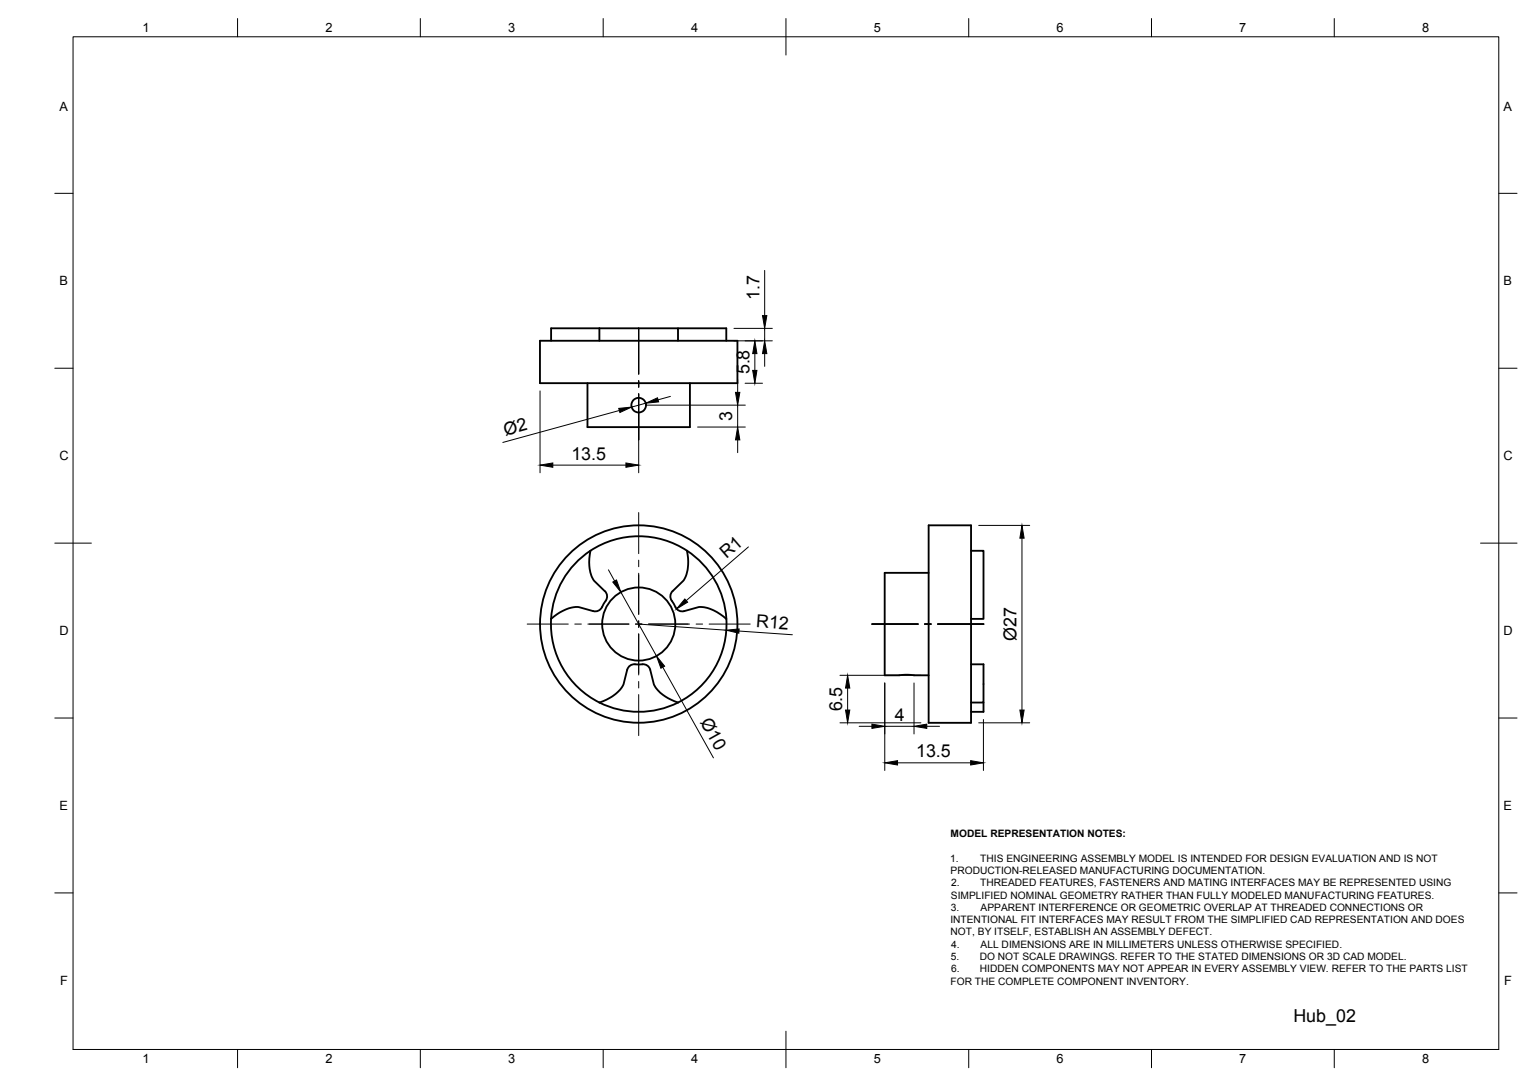
ISO-10303-21;
HEADER;
/* Generated by software containing ST-Developer
 * from STEP Tools, Inc. (www.steptools.com) 
 */

FILE_DESCRIPTION(
/* description */ (''),
/* implementation_level */ '2;1');

FILE_NAME(
/* name */ 'Hub_02.step',
/* time_stamp */ '2026-10-05T21:34:53-07:00',
/* author */ (''),
/* organization */ (''),
/* preprocessor_version */ 'ST-DEVELOPER v20.2',
/* originating_system */ 'Autodesk Translation Framework v15.15.0.0',
/* authorisation */ '');

FILE_SCHEMA (('AUTOMOTIVE_DESIGN { 1 0 10303 214 3 1 1 }'));
ENDSEC;

DATA;
#10=MECHANICAL_DESIGN_GEOMETRIC_PRESENTATION_REPRESENTATION('',(#67),#9822);
#49=SHAPE_REPRESENTATION_RELATIONSHIP('SRR','None',#9859,#58);
#58=ADVANCED_BREP_SHAPE_REPRESENTATION('',(#76),#9815);
#67=STYLED_ITEM('',(#9911),#76);
#76=MANIFOLD_SOLID_BREP('Body1',#3290);
#90=FACE_BOUND('',#562,.T.);
#91=FACE_BOUND('',#566,.T.);
#92=FACE_BOUND('',#568,.T.);
#93=FACE_BOUND('',#570,.T.);
#94=FACE_BOUND('',#573,.T.);
#138=B_SPLINE_CURVE_WITH_KNOTS('',3,(#9018,#9019,#9020,#9021,#9022,#9023,
#9024,#9025,#9026,#9027,#9028,#9029,#9030,#9031,#9032,#9033,#9034,#9035),
 .UNSPECIFIED.,.F.,.F.,(4,2,2,2,2,2,2,2,4),(0.,0.0377244205563716,0.0754488411127431,
0.113172721595804,0.150896602078865,0.188620482561925,0.226344363044986,
0.264068783601358,0.301793204157729),.UNSPECIFIED.);
#139=B_SPLINE_CURVE_WITH_KNOTS('',3,(#9036,#9037,#9038,#9039,#9040,#9041,
#9042,#9043,#9044,#9045,#9046,#9047,#9048,#9049,#9050,#9051,#9052,#9053),
 .UNSPECIFIED.,.F.,.F.,(4,2,2,2,2,2,2,2,4),(0.301793204157729,0.339517624714101,
0.377242045270472,0.414965925753533,0.452689806236594,0.490413686719655,
0.528137567202715,0.565861987759087,0.603586408315459),.UNSPECIFIED.);
#140=B_SPLINE_CURVE_WITH_KNOTS('',3,(#9074,#9075,#9076,#9077,#9078,#9079,
#9080,#9081,#9082,#9083,#9084,#9085,#9086,#9087,#9088,#9089,#9090,#9091),
 .UNSPECIFIED.,.F.,.F.,(4,2,2,2,2,2,2,2,4),(-0.302227736861757,-0.264448211272738,
-0.226668685683718,-0.188891277057298,-0.151113868430879,-0.113336459804459,
-0.0755590511780388,-0.0377795255890194,0.),.UNSPECIFIED.);
#141=B_SPLINE_CURVE_WITH_KNOTS('',3,(#9151,#9152,#9153,#9154,#9155,#9156,
#9157,#9158,#9159,#9160),.UNSPECIFIED.,.F.,.F.,(4,2,2,2,4),(-0.142515337525874,
-0.116550796129695,-0.0827833358062311,-0.0239794870259187,0.),
 .UNSPECIFIED.);
#142=B_SPLINE_CURVE_WITH_KNOTS('',3,(#9171,#9172,#9173,#9174,#9175,#9176,
#9177,#9178,#9179,#9180),.UNSPECIFIED.,.F.,.F.,(4,2,2,2,4),(-1.69587031053129,
-0.72373117069956,-0.441822634924292,-0.252830368936358,0.),
 .UNSPECIFIED.);
#143=B_SPLINE_CURVE_WITH_KNOTS('',3,(#9182,#9183,#9184,#9185,#9186,#9187,
#9188,#9189,#9190,#9191),.UNSPECIFIED.,.F.,.F.,(4,2,2,2,4),(-0.142515337583282,
-0.116550796158019,-0.0827833358058086,-0.0239794870257561,0.),
 .UNSPECIFIED.);
#144=B_SPLINE_CURVE_WITH_KNOTS('',3,(#9202,#9203,#9204,#9205,#9206,#9207,
#9208,#9209,#9210,#9211),.UNSPECIFIED.,.F.,.F.,(4,2,2,2,4),(-1.69587031141743,
-0.723731170975569,-0.441822635061051,-0.252830368989318,0.),
 .UNSPECIFIED.);
#145=B_SPLINE_CURVE_WITH_KNOTS('',3,(#9213,#9214,#9215,#9216,#9217,#9218,
#9219,#9220,#9221,#9222),.UNSPECIFIED.,.F.,.F.,(4,2,2,2,4),(-0.142515337540036,
-0.116550796137795,-0.0827833358078941,-0.0239794870259568,0.),
 .UNSPECIFIED.);
#146=B_SPLINE_CURVE_WITH_KNOTS('',3,(#9233,#9234,#9235,#9236,#9237,#9238,
#9239,#9240,#9241,#9242),.UNSPECIFIED.,.F.,.F.,(4,2,2,2,4),(-1.69587030996743,
-0.72373117051105,-0.441822634822492,-0.252830368895713,0.),
 .UNSPECIFIED.);
#147=B_SPLINE_CURVE_WITH_KNOTS('',3,(#9289,#9290,#9291,#9292,#9293,#9294,
#9295,#9296,#9297,#9298),.UNSPECIFIED.,.F.,.F.,(4,2,2,2,4),(-0.142515337540036,
-0.116550796137795,-0.0827833358078941,-0.0239794870259568,0.),
 .UNSPECIFIED.);
#148=B_SPLINE_CURVE_WITH_KNOTS('',3,(#9321,#9322,#9323,#9324,#9325,#9326,
#9327,#9328,#9329,#9330),.UNSPECIFIED.,.F.,.F.,(4,2,2,2,4),(-1.69587030996743,
-0.72373117051105,-0.441822634822492,-0.252830368895713,0.),
 .UNSPECIFIED.);
#149=B_SPLINE_CURVE_WITH_KNOTS('',3,(#9372,#9373,#9374,#9375,#9376,#9377,
#9378,#9379,#9380,#9381),.UNSPECIFIED.,.F.,.F.,(4,2,2,2,4),(-0.142515337583282,
-0.116550796158019,-0.0827833358058086,-0.0239794870257561,0.),
 .UNSPECIFIED.);
#150=B_SPLINE_CURVE_WITH_KNOTS('',3,(#9404,#9405,#9406,#9407,#9408,#9409,
#9410,#9411,#9412,#9413),.UNSPECIFIED.,.F.,.F.,(4,2,2,2,4),(-1.69587031141743,
-0.723731170975569,-0.441822635061051,-0.252830368989318,0.),
 .UNSPECIFIED.);
#151=B_SPLINE_CURVE_WITH_KNOTS('',3,(#9457,#9458,#9459,#9460,#9461,#9462,
#9463,#9464,#9465,#9466),.UNSPECIFIED.,.F.,.F.,(4,2,2,2,4),(-0.142515337525874,
-0.116550796129695,-0.0827833358062311,-0.0239794870259187,0.),
 .UNSPECIFIED.);
#152=B_SPLINE_CURVE_WITH_KNOTS('',3,(#9493,#9494,#9495,#9496,#9497,#9498,
#9499,#9500,#9501,#9502),.UNSPECIFIED.,.F.,.F.,(4,2,2,2,4),(-1.69587031053129,
-0.72373117069956,-0.441822634924292,-0.252830368936358,0.),
 .UNSPECIFIED.);
#175=B_SPLINE_SURFACE_WITH_KNOTS('',3,1,((#9269,#9270),(#9271,#9272),(#9273,
#9274),(#9275,#9276),(#9277,#9278),(#9279,#9280),(#9281,#9282),(#9283,#9284),
(#9285,#9286),(#9287,#9288)),.UNSPECIFIED.,.F.,.F.,.F.,(4,2,2,2,4),(2,2),
(-0.142515337540036,-0.116550796137795,-0.0827833358078941,-0.0239794870259568,
0.),(0.,0.78),.UNSPECIFIED.);
#176=B_SPLINE_SURFACE_WITH_KNOTS('',3,1,((#9299,#9300),(#9301,#9302),(#9303,
#9304),(#9305,#9306),(#9307,#9308),(#9309,#9310),(#9311,#9312),(#9313,#9314),
(#9315,#9316),(#9317,#9318)),.UNSPECIFIED.,.F.,.F.,.F.,(4,2,2,2,4),(2,2),
(-1.69587030996743,-0.72373117051105,-0.441822634822492,-0.252830368895713,
0.),(0.,0.78),.UNSPECIFIED.);
#177=B_SPLINE_SURFACE_WITH_KNOTS('',3,1,((#9352,#9353),(#9354,#9355),(#9356,
#9357),(#9358,#9359),(#9360,#9361),(#9362,#9363),(#9364,#9365),(#9366,#9367),
(#9368,#9369),(#9370,#9371)),.UNSPECIFIED.,.F.,.F.,.F.,(4,2,2,2,4),(2,2),
(-0.142515337583282,-0.116550796158019,-0.0827833358058086,-0.0239794870257561,
0.),(0.,0.78),.UNSPECIFIED.);
#178=B_SPLINE_SURFACE_WITH_KNOTS('',3,1,((#9382,#9383),(#9384,#9385),(#9386,
#9387),(#9388,#9389),(#9390,#9391),(#9392,#9393),(#9394,#9395),(#9396,#9397),
(#9398,#9399),(#9400,#9401)),.UNSPECIFIED.,.F.,.F.,.F.,(4,2,2,2,4),(2,2),
(-1.69587031141743,-0.723731170975569,-0.441822635061051,-0.252830368989318,
0.),(0.,0.78),.UNSPECIFIED.);
#179=B_SPLINE_SURFACE_WITH_KNOTS('',3,1,((#9435,#9436),(#9437,#9438),(#9439,
#9440),(#9441,#9442),(#9443,#9444),(#9445,#9446),(#9447,#9448),(#9449,#9450),
(#9451,#9452),(#9453,#9454)),.UNSPECIFIED.,.F.,.F.,.F.,(4,2,2,2,4),(2,2),
(-0.142515337525874,-0.116550796129695,-0.0827833358062311,-0.0239794870259187,
0.),(0.,0.78),.UNSPECIFIED.);
#180=B_SPLINE_SURFACE_WITH_KNOTS('',3,1,((#9471,#9472),(#9473,#9474),(#9475,
#9476),(#9477,#9478),(#9479,#9480),(#9481,#9482),(#9483,#9484),(#9485,#9486),
(#9487,#9488),(#9489,#9490)),.UNSPECIFIED.,.F.,.F.,.F.,(4,2,2,2,4),(2,2),
(-1.69587031053129,-0.72373117069956,-0.441822634924292,-0.252830368936358,
0.),(0.,0.78),.UNSPECIFIED.);
#212=PLANE('',#3570);
#213=PLANE('',#3571);
#214=PLANE('',#3573);
#215=PLANE('',#3575);
#216=PLANE('',#3589);
#217=PLANE('',#3598);
#218=PLANE('',#3611);
#219=PLANE('',#3614);
#220=PLANE('',#3619);
#221=PLANE('',#3620);
#222=PLANE('',#3623);
#223=PLANE('',#3628);
#224=PLANE('',#3629);
#225=PLANE('',#3632);
#226=PLANE('',#3637);
#227=PLANE('',#3640);
#228=PLANE('',#3643);
#359=FACE_OUTER_BOUND('',#551,.T.);
#360=FACE_OUTER_BOUND('',#552,.T.);
#361=FACE_OUTER_BOUND('',#553,.T.);
#362=FACE_OUTER_BOUND('',#554,.T.);
#363=FACE_OUTER_BOUND('',#555,.T.);
#364=FACE_OUTER_BOUND('',#556,.T.);
#365=FACE_OUTER_BOUND('',#557,.T.);
#366=FACE_OUTER_BOUND('',#558,.T.);
#367=FACE_OUTER_BOUND('',#559,.T.);
#368=FACE_OUTER_BOUND('',#560,.T.);
#369=FACE_OUTER_BOUND('',#561,.T.);
#370=FACE_OUTER_BOUND('',#563,.T.);
#371=FACE_OUTER_BOUND('',#564,.T.);
#372=FACE_OUTER_BOUND('',#565,.T.);
#373=FACE_OUTER_BOUND('',#567,.T.);
#374=FACE_OUTER_BOUND('',#569,.T.);
#375=FACE_OUTER_BOUND('',#571,.T.);
#376=FACE_OUTER_BOUND('',#572,.T.);
#377=FACE_OUTER_BOUND('',#574,.T.);
#378=FACE_OUTER_BOUND('',#575,.T.);
#379=FACE_OUTER_BOUND('',#576,.T.);
#380=FACE_OUTER_BOUND('',#577,.T.);
#381=FACE_OUTER_BOUND('',#578,.T.);
#382=FACE_OUTER_BOUND('',#579,.T.);
#383=FACE_OUTER_BOUND('',#580,.T.);
#384=FACE_OUTER_BOUND('',#581,.T.);
#385=FACE_OUTER_BOUND('',#582,.T.);
#386=FACE_OUTER_BOUND('',#583,.T.);
#387=FACE_OUTER_BOUND('',#584,.T.);
#388=FACE_OUTER_BOUND('',#585,.T.);
#389=FACE_OUTER_BOUND('',#586,.T.);
#390=FACE_OUTER_BOUND('',#587,.T.);
#391=FACE_OUTER_BOUND('',#588,.T.);
#392=FACE_OUTER_BOUND('',#589,.T.);
#393=FACE_OUTER_BOUND('',#590,.T.);
#394=FACE_OUTER_BOUND('',#591,.T.);
#395=FACE_OUTER_BOUND('',#592,.T.);
#396=FACE_OUTER_BOUND('',#593,.T.);
#397=FACE_OUTER_BOUND('',#594,.T.);
#398=FACE_OUTER_BOUND('',#595,.T.);
#399=FACE_OUTER_BOUND('',#596,.T.);
#400=FACE_OUTER_BOUND('',#597,.T.);
#401=FACE_OUTER_BOUND('',#598,.T.);
#551=EDGE_LOOP('',(#2610,#2611,#2612,#2613,#2614,#2615));
#552=EDGE_LOOP('',(#2616,#2617,#2618,#2619));
#553=EDGE_LOOP('',(#2620,#2621,#2622,#2623));
#554=EDGE_LOOP('',(#2624,#2625,#2626,#2627,#2628));
#555=EDGE_LOOP('',(#2629,#2630,#2631,#2632));
#556=EDGE_LOOP('',(#2633,#2634,#2635,#2636,#2637));
#557=EDGE_LOOP('',(#2638,#2639,#2640,#2641,#2642,#2643,#2644,#2645));
#558=EDGE_LOOP('',(#2646,#2647,#2648,#2649));
#559=EDGE_LOOP('',(#2650,#2651,#2652,#2653));
#560=EDGE_LOOP('',(#2654,#2655,#2656,#2657));
#561=EDGE_LOOP('',(#2658));
#562=EDGE_LOOP('',(#2659,#2660,#2661,#2662,#2663,#2664));
#563=EDGE_LOOP('',(#2665,#2666,#2667,#2668));
#564=EDGE_LOOP('',(#2669,#2670,#2671,#2672));
#565=EDGE_LOOP('',(#2673,#2674,#2675,#2676,#2677,#2678,#2679,#2680,#2681,
#2682,#2683,#2684,#2685,#2686,#2687,#2688,#2689,#2690,#2691,#2692,#2693,
#2694,#2695,#2696));
#566=EDGE_LOOP('',(#2697));
#567=EDGE_LOOP('',(#2698,#2699,#2700,#2701));
#568=EDGE_LOOP('',(#2702,#2703));
#569=EDGE_LOOP('',(#2704));
#570=EDGE_LOOP('',(#2705,#2706,#2707,#2708,#2709));
#571=EDGE_LOOP('',(#2710,#2711,#2712,#2713));
#572=EDGE_LOOP('',(#2714));
#573=EDGE_LOOP('',(#2715));
#574=EDGE_LOOP('',(#2716,#2717,#2718,#2719));
#575=EDGE_LOOP('',(#2720,#2721,#2722,#2723));
#576=EDGE_LOOP('',(#2724,#2725,#2726,#2727));
#577=EDGE_LOOP('',(#2728,#2729,#2730,#2731,#2732));
#578=EDGE_LOOP('',(#2733,#2734,#2735,#2736,#2737));
#579=EDGE_LOOP('',(#2738,#2739,#2740,#2741));
#580=EDGE_LOOP('',(#2742,#2743,#2744,#2745));
#581=EDGE_LOOP('',(#2746,#2747,#2748,#2749,#2750,#2751,#2752,#2753));
#582=EDGE_LOOP('',(#2754,#2755,#2756,#2757));
#583=EDGE_LOOP('',(#2758,#2759,#2760,#2761));
#584=EDGE_LOOP('',(#2762,#2763,#2764,#2765));
#585=EDGE_LOOP('',(#2766,#2767,#2768,#2769,#2770));
#586=EDGE_LOOP('',(#2771,#2772,#2773,#2774,#2775));
#587=EDGE_LOOP('',(#2776,#2777,#2778,#2779));
#588=EDGE_LOOP('',(#2780,#2781,#2782,#2783));
#589=EDGE_LOOP('',(#2784,#2785,#2786,#2787,#2788,#2789,#2790,#2791));
#590=EDGE_LOOP('',(#2792,#2793,#2794,#2795));
#591=EDGE_LOOP('',(#2796,#2797,#2798,#2799));
#592=EDGE_LOOP('',(#2800,#2801,#2802,#2803));
#593=EDGE_LOOP('',(#2804,#2805,#2806,#2807,#2808));
#594=EDGE_LOOP('',(#2809,#2810,#2811,#2812));
#595=EDGE_LOOP('',(#2813,#2814,#2815,#2816,#2817));
#596=EDGE_LOOP('',(#2818,#2819,#2820,#2821));
#597=EDGE_LOOP('',(#2822,#2823,#2824,#2825));
#598=EDGE_LOOP('',(#2826,#2827,#2828,#2829,#2830,#2831,#2832,#2833));
#781=LINE('',#9016,#1040);
#782=LINE('',#9056,#1041);
#783=LINE('',#9058,#1042);
#784=LINE('',#9059,#1043);
#785=LINE('',#9062,#1044);
#786=LINE('',#9065,#1045);
#787=LINE('',#9068,#1046);
#788=LINE('',#9070,#1047);
#789=LINE('',#9071,#1048);
#790=LINE('',#9092,#1049);
#791=LINE('',#9095,#1050);
#792=LINE('',#9096,#1051);
#793=LINE('',#9101,#1052);
#794=LINE('',#9107,#1053);
#795=LINE('',#9111,#1054);
#796=LINE('',#9116,#1055);
#797=LINE('',#9120,#1056);
#798=LINE('',#9125,#1057);
#799=LINE('',#9129,#1058);
#800=LINE('',#9139,#1059);
#801=LINE('',#9142,#1060);
#802=LINE('',#9145,#1061);
#803=LINE('',#9148,#1062);
#804=LINE('',#9162,#1063);
#805=LINE('',#9170,#1064);
#806=LINE('',#9193,#1065);
#807=LINE('',#9201,#1066);
#808=LINE('',#9224,#1067);
#809=LINE('',#9232,#1068);
#810=LINE('',#9247,#1069);
#811=LINE('',#9252,#1070);
#812=LINE('',#9257,#1071);
#813=LINE('',#9260,#1072);
#814=LINE('',#9263,#1073);
#815=LINE('',#9267,#1074);
#816=LINE('',#9268,#1075);
#817=LINE('',#9320,#1076);
#818=LINE('',#9333,#1077);
#819=LINE('',#9334,#1078);
#820=LINE('',#9340,#1079);
#821=LINE('',#9343,#1080);
#822=LINE('',#9346,#1081);
#823=LINE('',#9350,#1082);
#824=LINE('',#9351,#1083);
#825=LINE('',#9403,#1084);
#826=LINE('',#9416,#1085);
#827=LINE('',#9417,#1086);
#828=LINE('',#9423,#1087);
#829=LINE('',#9426,#1088);
#830=LINE('',#9429,#1089);
#831=LINE('',#9433,#1090);
#832=LINE('',#9434,#1091);
#833=LINE('',#9456,#1092);
#834=LINE('',#9469,#1093);
#835=LINE('',#9492,#1094);
#836=LINE('',#9505,#1095);
#837=LINE('',#9506,#1096);
#1040=VECTOR('',#4203,1.);
#1041=VECTOR('',#4206,10.);
#1042=VECTOR('',#4207,10.);
#1043=VECTOR('',#4208,10.);
#1044=VECTOR('',#4211,10.);
#1045=VECTOR('',#4214,10.);
#1046=VECTOR('',#4217,10.);
#1047=VECTOR('',#4218,10.);
#1048=VECTOR('',#4219,10.);
#1049=VECTOR('',#4222,10.);
#1050=VECTOR('',#4225,10.);
#1051=VECTOR('',#4226,10.);
#1052=VECTOR('',#4231,5.);
#1053=VECTOR('',#4238,10.);
#1054=VECTOR('',#4241,10.);
#1055=VECTOR('',#4246,10.);
#1056=VECTOR('',#4249,10.);
#1057=VECTOR('',#4254,10.);
#1058=VECTOR('',#4257,10.);
#1059=VECTOR('',#4272,10.);
#1060=VECTOR('',#4275,10.);
#1061=VECTOR('',#4278,10.);
#1062=VECTOR('',#4281,10.);
#1063=VECTOR('',#4284,10.);
#1064=VECTOR('',#4291,10.);
#1065=VECTOR('',#4292,10.);
#1066=VECTOR('',#4299,10.);
#1067=VECTOR('',#4300,10.);
#1068=VECTOR('',#4307,10.);
#1069=VECTOR('',#4312,7.);
#1070=VECTOR('',#4319,13.5);
#1071=VECTOR('',#4326,10.);
#1072=VECTOR('',#4329,10.);
#1073=VECTOR('',#4332,10.);
#1074=VECTOR('',#4337,10.);
#1075=VECTOR('',#4338,10.);
#1076=VECTOR('',#4339,10.);
#1077=VECTOR('',#4342,10.);
#1078=VECTOR('',#4343,10.);
#1079=VECTOR('',#4352,10.);
#1080=VECTOR('',#4355,10.);
#1081=VECTOR('',#4358,10.);
#1082=VECTOR('',#4363,10.);
#1083=VECTOR('',#4364,10.);
#1084=VECTOR('',#4365,10.);
#1085=VECTOR('',#4368,10.);
#1086=VECTOR('',#4369,10.);
#1087=VECTOR('',#4378,10.);
#1088=VECTOR('',#4381,10.);
#1089=VECTOR('',#4384,10.);
#1090=VECTOR('',#4389,10.);
#1091=VECTOR('',#4390,10.);
#1092=VECTOR('',#4391,10.);
#1093=VECTOR('',#4394,10.);
#1094=VECTOR('',#4397,10.);
#1095=VECTOR('',#4400,10.);
#1096=VECTOR('',#4401,10.);
#1259=CIRCLE('',#3568,1.);
#1260=CIRCLE('',#3569,1.);
#1261=CIRCLE('',#3572,1.);
#1262=CIRCLE('',#3577,5.);
#1263=CIRCLE('',#3578,5.);
#1264=CIRCLE('',#3579,5.);
#1265=CIRCLE('',#3581,12.);
#1266=CIRCLE('',#3582,12.);
#1267=CIRCLE('',#3584,12.);
#1268=CIRCLE('',#3585,12.);
#1269=CIRCLE('',#3587,12.);
#1270=CIRCLE('',#3588,12.);
#1271=CIRCLE('',#3590,13.5);
#1272=CIRCLE('',#3591,12.);
#1273=CIRCLE('',#3592,12.);
#1274=CIRCLE('',#3593,12.);
#1275=CIRCLE('',#3595,12.);
#1276=CIRCLE('',#3597,12.);
#1277=CIRCLE('',#3599,1.);
#1278=CIRCLE('',#3600,5.529);
#1279=CIRCLE('',#3601,1.);
#1280=CIRCLE('',#3602,1.);
#1281=CIRCLE('',#3603,5.529);
#1282=CIRCLE('',#3604,1.);
#1283=CIRCLE('',#3605,1.);
#1284=CIRCLE('',#3606,5.529);
#1285=CIRCLE('',#3607,1.);
#1286=CIRCLE('',#3609,7.);
#1287=CIRCLE('',#3610,7.);
#1288=CIRCLE('',#3613,13.5);
#1289=CIRCLE('',#3616,5.529);
#1290=CIRCLE('',#3618,1.);
#1291=CIRCLE('',#3622,1.);
#1292=CIRCLE('',#3625,5.529);
#1293=CIRCLE('',#3627,1.);
#1294=CIRCLE('',#3631,1.);
#1295=CIRCLE('',#3634,5.529);
#1296=CIRCLE('',#3636,1.);
#1297=CIRCLE('',#3639,12.);
#1298=CIRCLE('',#3642,1.);
#1489=VERTEX_POINT('',#9011);
#1490=VERTEX_POINT('',#9012);
#1491=VERTEX_POINT('',#9015);
#1492=VERTEX_POINT('',#9017);
#1493=VERTEX_POINT('',#9055);
#1494=VERTEX_POINT('',#9057);
#1495=VERTEX_POINT('',#9061);
#1496=VERTEX_POINT('',#9063);
#1497=VERTEX_POINT('',#9067);
#1498=VERTEX_POINT('',#9069);
#1499=VERTEX_POINT('',#9073);
#1500=VERTEX_POINT('',#9094);
#1501=VERTEX_POINT('',#9098);
#1502=VERTEX_POINT('',#9100);
#1503=VERTEX_POINT('',#9105);
#1504=VERTEX_POINT('',#9106);
#1505=VERTEX_POINT('',#9108);
#1506=VERTEX_POINT('',#9110);
#1507=VERTEX_POINT('',#9114);
#1508=VERTEX_POINT('',#9115);
#1509=VERTEX_POINT('',#9117);
#1510=VERTEX_POINT('',#9119);
#1511=VERTEX_POINT('',#9123);
#1512=VERTEX_POINT('',#9124);
#1513=VERTEX_POINT('',#9126);
#1514=VERTEX_POINT('',#9128);
#1515=VERTEX_POINT('',#9132);
#1516=VERTEX_POINT('',#9138);
#1517=VERTEX_POINT('',#9140);
#1518=VERTEX_POINT('',#9144);
#1519=VERTEX_POINT('',#9146);
#1520=VERTEX_POINT('',#9150);
#1521=VERTEX_POINT('',#9161);
#1522=VERTEX_POINT('',#9163);
#1523=VERTEX_POINT('',#9165);
#1524=VERTEX_POINT('',#9167);
#1525=VERTEX_POINT('',#9169);
#1526=VERTEX_POINT('',#9181);
#1527=VERTEX_POINT('',#9192);
#1528=VERTEX_POINT('',#9194);
#1529=VERTEX_POINT('',#9196);
#1530=VERTEX_POINT('',#9198);
#1531=VERTEX_POINT('',#9200);
#1532=VERTEX_POINT('',#9212);
#1533=VERTEX_POINT('',#9223);
#1534=VERTEX_POINT('',#9225);
#1535=VERTEX_POINT('',#9227);
#1536=VERTEX_POINT('',#9229);
#1537=VERTEX_POINT('',#9231);
#1538=VERTEX_POINT('',#9244);
#1539=VERTEX_POINT('',#9246);
#1540=VERTEX_POINT('',#9251);
#1541=VERTEX_POINT('',#9256);
#1542=VERTEX_POINT('',#9258);
#1543=VERTEX_POINT('',#9262);
#1544=VERTEX_POINT('',#9266);
#1545=VERTEX_POINT('',#9319);
#1546=VERTEX_POINT('',#9332);
#1547=VERTEX_POINT('',#9339);
#1548=VERTEX_POINT('',#9341);
#1549=VERTEX_POINT('',#9345);
#1550=VERTEX_POINT('',#9349);
#1551=VERTEX_POINT('',#9402);
#1552=VERTEX_POINT('',#9415);
#1553=VERTEX_POINT('',#9422);
#1554=VERTEX_POINT('',#9424);
#1555=VERTEX_POINT('',#9428);
#1556=VERTEX_POINT('',#9432);
#1557=VERTEX_POINT('',#9455);
#1558=VERTEX_POINT('',#9468);
#1559=VERTEX_POINT('',#9491);
#1560=VERTEX_POINT('',#9504);
#1884=EDGE_CURVE('',#1489,#1490,#1259,.T.);
#1885=EDGE_CURVE('',#1490,#1489,#1260,.T.);
#1886=EDGE_CURVE('',#1490,#1491,#781,.T.);
#1887=EDGE_CURVE('',#1492,#1491,#138,.T.);
#1888=EDGE_CURVE('',#1491,#1492,#139,.T.);
#1889=EDGE_CURVE('',#1489,#1493,#782,.T.);
#1890=EDGE_CURVE('',#1494,#1493,#783,.T.);
#1891=EDGE_CURVE('',#1494,#1490,#784,.T.);
#1892=EDGE_CURVE('',#1490,#1495,#785,.T.);
#1893=EDGE_CURVE('',#1495,#1496,#1261,.T.);
#1894=EDGE_CURVE('',#1496,#1489,#786,.T.);
#1895=EDGE_CURVE('',#1493,#1497,#787,.T.);
#1896=EDGE_CURVE('',#1498,#1496,#788,.T.);
#1897=EDGE_CURVE('',#1497,#1498,#789,.T.);
#1898=EDGE_CURVE('',#1498,#1499,#140,.T.);
#1899=EDGE_CURVE('',#1499,#1495,#790,.T.);
#1900=EDGE_CURVE('',#1500,#1494,#791,.T.);
#1901=EDGE_CURVE('',#1499,#1500,#792,.T.);
#1902=EDGE_CURVE('',#1500,#1501,#1262,.T.);
#1903=EDGE_CURVE('',#1501,#1502,#793,.T.);
#1904=EDGE_CURVE('',#1502,#1502,#1263,.T.);
#1905=EDGE_CURVE('',#1501,#1497,#1264,.T.);
#1906=EDGE_CURVE('',#1503,#1504,#794,.T.);
#1907=EDGE_CURVE('',#1504,#1505,#1265,.T.);
#1908=EDGE_CURVE('',#1506,#1505,#795,.T.);
#1909=EDGE_CURVE('',#1506,#1503,#1266,.T.);
#1910=EDGE_CURVE('',#1507,#1508,#796,.T.);
#1911=EDGE_CURVE('',#1507,#1509,#1267,.T.);
#1912=EDGE_CURVE('',#1509,#1510,#797,.T.);
#1913=EDGE_CURVE('',#1510,#1508,#1268,.T.);
#1914=EDGE_CURVE('',#1511,#1512,#798,.T.);
#1915=EDGE_CURVE('',#1511,#1513,#1269,.T.);
#1916=EDGE_CURVE('',#1513,#1514,#799,.T.);
#1917=EDGE_CURVE('',#1514,#1512,#1270,.T.);
#1918=EDGE_CURVE('',#1515,#1515,#1271,.T.);
#1919=EDGE_CURVE('',#1514,#1508,#1272,.T.);
#1920=EDGE_CURVE('',#1510,#1505,#1273,.T.);
#1921=EDGE_CURVE('',#1504,#1512,#1274,.T.);
#1922=EDGE_CURVE('',#1514,#1516,#800,.T.);
#1923=EDGE_CURVE('',#1516,#1517,#1275,.T.);
#1924=EDGE_CURVE('',#1508,#1517,#801,.T.);
#1925=EDGE_CURVE('',#1510,#1518,#802,.T.);
#1926=EDGE_CURVE('',#1518,#1519,#1276,.T.);
#1927=EDGE_CURVE('',#1505,#1519,#803,.T.);
#1928=EDGE_CURVE('',#1511,#1520,#141,.T.);
#1929=EDGE_CURVE('',#1520,#1521,#804,.T.);
#1930=EDGE_CURVE('',#1522,#1521,#1277,.T.);
#1931=EDGE_CURVE('',#1522,#1523,#1278,.T.);
#1932=EDGE_CURVE('',#1524,#1523,#1279,.T.);
#1933=EDGE_CURVE('',#1524,#1525,#805,.T.);
#1934=EDGE_CURVE('',#1525,#1503,#142,.T.);
#1935=EDGE_CURVE('',#1506,#1526,#143,.T.);
#1936=EDGE_CURVE('',#1526,#1527,#806,.T.);
#1937=EDGE_CURVE('',#1528,#1527,#1280,.T.);
#1938=EDGE_CURVE('',#1528,#1529,#1281,.T.);
#1939=EDGE_CURVE('',#1530,#1529,#1282,.T.);
#1940=EDGE_CURVE('',#1530,#1531,#807,.T.);
#1941=EDGE_CURVE('',#1531,#1509,#144,.T.);
#1942=EDGE_CURVE('',#1507,#1532,#145,.T.);
#1943=EDGE_CURVE('',#1532,#1533,#808,.T.);
#1944=EDGE_CURVE('',#1534,#1533,#1283,.T.);
#1945=EDGE_CURVE('',#1534,#1535,#1284,.T.);
#1946=EDGE_CURVE('',#1536,#1535,#1285,.T.);
#1947=EDGE_CURVE('',#1536,#1537,#809,.T.);
#1948=EDGE_CURVE('',#1537,#1513,#146,.T.);
#1949=EDGE_CURVE('',#1538,#1538,#1286,.F.);
#1950=EDGE_CURVE('',#1538,#1539,#810,.T.);
#1951=EDGE_CURVE('',#1539,#1539,#1287,.T.);
#1952=EDGE_CURVE('',#1515,#1540,#811,.T.);
#1953=EDGE_CURVE('',#1540,#1540,#1288,.T.);
#1954=EDGE_CURVE('',#1534,#1541,#812,.T.);
#1955=EDGE_CURVE('',#1541,#1542,#1289,.T.);
#1956=EDGE_CURVE('',#1535,#1542,#813,.T.);
#1957=EDGE_CURVE('',#1533,#1543,#814,.T.);
#1958=EDGE_CURVE('',#1543,#1541,#1290,.T.);
#1959=EDGE_CURVE('',#1532,#1544,#815,.T.);
#1960=EDGE_CURVE('',#1544,#1543,#816,.T.);
#1961=EDGE_CURVE('',#1517,#1544,#147,.T.);
#1962=EDGE_CURVE('',#1537,#1545,#817,.T.);
#1963=EDGE_CURVE('',#1545,#1516,#148,.T.);
#1964=EDGE_CURVE('',#1536,#1546,#818,.T.);
#1965=EDGE_CURVE('',#1546,#1545,#819,.T.);
#1966=EDGE_CURVE('',#1542,#1546,#1291,.T.);
#1967=EDGE_CURVE('',#1528,#1547,#820,.T.);
#1968=EDGE_CURVE('',#1547,#1548,#1292,.T.);
#1969=EDGE_CURVE('',#1529,#1548,#821,.T.);
#1970=EDGE_CURVE('',#1527,#1549,#822,.T.);
#1971=EDGE_CURVE('',#1549,#1547,#1293,.T.);
#1972=EDGE_CURVE('',#1526,#1550,#823,.T.);
#1973=EDGE_CURVE('',#1550,#1549,#824,.T.);
#1974=EDGE_CURVE('',#1519,#1550,#149,.T.);
#1975=EDGE_CURVE('',#1531,#1551,#825,.T.);
#1976=EDGE_CURVE('',#1551,#1518,#150,.T.);
#1977=EDGE_CURVE('',#1530,#1552,#826,.T.);
#1978=EDGE_CURVE('',#1552,#1551,#827,.T.);
#1979=EDGE_CURVE('',#1548,#1552,#1294,.T.);
#1980=EDGE_CURVE('',#1522,#1553,#828,.T.);
#1981=EDGE_CURVE('',#1553,#1554,#1295,.T.);
#1982=EDGE_CURVE('',#1523,#1554,#829,.T.);
#1983=EDGE_CURVE('',#1521,#1555,#830,.T.);
#1984=EDGE_CURVE('',#1555,#1553,#1296,.T.);
#1985=EDGE_CURVE('',#1520,#1556,#831,.T.);
#1986=EDGE_CURVE('',#1556,#1555,#832,.T.);
#1987=EDGE_CURVE('',#1512,#1557,#833,.T.);
#1988=EDGE_CURVE('',#1557,#1556,#151,.T.);
#1989=EDGE_CURVE('',#1504,#1558,#834,.T.);
#1990=EDGE_CURVE('',#1558,#1557,#1297,.T.);
#1991=EDGE_CURVE('',#1525,#1559,#835,.T.);
#1992=EDGE_CURVE('',#1559,#1558,#152,.T.);
#1993=EDGE_CURVE('',#1524,#1560,#836,.T.);
#1994=EDGE_CURVE('',#1560,#1559,#837,.T.);
#1995=EDGE_CURVE('',#1554,#1560,#1298,.T.);
#2610=ORIENTED_EDGE('',*,*,#1884,.F.);
#2611=ORIENTED_EDGE('',*,*,#1885,.F.);
#2612=ORIENTED_EDGE('',*,*,#1886,.T.);
#2613=ORIENTED_EDGE('',*,*,#1887,.F.);
#2614=ORIENTED_EDGE('',*,*,#1888,.F.);
#2615=ORIENTED_EDGE('',*,*,#1886,.F.);
#2616=ORIENTED_EDGE('',*,*,#1885,.T.);
#2617=ORIENTED_EDGE('',*,*,#1889,.T.);
#2618=ORIENTED_EDGE('',*,*,#1890,.F.);
#2619=ORIENTED_EDGE('',*,*,#1891,.T.);
#2620=ORIENTED_EDGE('',*,*,#1884,.T.);
#2621=ORIENTED_EDGE('',*,*,#1892,.T.);
#2622=ORIENTED_EDGE('',*,*,#1893,.T.);
#2623=ORIENTED_EDGE('',*,*,#1894,.T.);
#2624=ORIENTED_EDGE('',*,*,#1895,.F.);
#2625=ORIENTED_EDGE('',*,*,#1889,.F.);
#2626=ORIENTED_EDGE('',*,*,#1894,.F.);
#2627=ORIENTED_EDGE('',*,*,#1896,.F.);
#2628=ORIENTED_EDGE('',*,*,#1897,.F.);
#2629=ORIENTED_EDGE('',*,*,#1898,.F.);
#2630=ORIENTED_EDGE('',*,*,#1896,.T.);
#2631=ORIENTED_EDGE('',*,*,#1893,.F.);
#2632=ORIENTED_EDGE('',*,*,#1899,.F.);
#2633=ORIENTED_EDGE('',*,*,#1900,.F.);
#2634=ORIENTED_EDGE('',*,*,#1901,.F.);
#2635=ORIENTED_EDGE('',*,*,#1899,.T.);
#2636=ORIENTED_EDGE('',*,*,#1892,.F.);
#2637=ORIENTED_EDGE('',*,*,#1891,.F.);
#2638=ORIENTED_EDGE('',*,*,#1902,.T.);
#2639=ORIENTED_EDGE('',*,*,#1903,.T.);
#2640=ORIENTED_EDGE('',*,*,#1904,.F.);
#2641=ORIENTED_EDGE('',*,*,#1903,.F.);
#2642=ORIENTED_EDGE('',*,*,#1905,.T.);
#2643=ORIENTED_EDGE('',*,*,#1897,.T.);
#2644=ORIENTED_EDGE('',*,*,#1898,.T.);
#2645=ORIENTED_EDGE('',*,*,#1901,.T.);
#2646=ORIENTED_EDGE('',*,*,#1906,.T.);
#2647=ORIENTED_EDGE('',*,*,#1907,.T.);
#2648=ORIENTED_EDGE('',*,*,#1908,.F.);
#2649=ORIENTED_EDGE('',*,*,#1909,.T.);
#2650=ORIENTED_EDGE('',*,*,#1910,.F.);
#2651=ORIENTED_EDGE('',*,*,#1911,.T.);
#2652=ORIENTED_EDGE('',*,*,#1912,.T.);
#2653=ORIENTED_EDGE('',*,*,#1913,.T.);
#2654=ORIENTED_EDGE('',*,*,#1914,.F.);
#2655=ORIENTED_EDGE('',*,*,#1915,.T.);
#2656=ORIENTED_EDGE('',*,*,#1916,.T.);
#2657=ORIENTED_EDGE('',*,*,#1917,.T.);
#2658=ORIENTED_EDGE('',*,*,#1918,.F.);
#2659=ORIENTED_EDGE('',*,*,#1919,.T.);
#2660=ORIENTED_EDGE('',*,*,#1913,.F.);
#2661=ORIENTED_EDGE('',*,*,#1920,.T.);
#2662=ORIENTED_EDGE('',*,*,#1907,.F.);
#2663=ORIENTED_EDGE('',*,*,#1921,.T.);
#2664=ORIENTED_EDGE('',*,*,#1917,.F.);
#2665=ORIENTED_EDGE('',*,*,#1919,.F.);
#2666=ORIENTED_EDGE('',*,*,#1922,.T.);
#2667=ORIENTED_EDGE('',*,*,#1923,.T.);
#2668=ORIENTED_EDGE('',*,*,#1924,.F.);
#2669=ORIENTED_EDGE('',*,*,#1920,.F.);
#2670=ORIENTED_EDGE('',*,*,#1925,.T.);
#2671=ORIENTED_EDGE('',*,*,#1926,.T.);
#2672=ORIENTED_EDGE('',*,*,#1927,.F.);
#2673=ORIENTED_EDGE('',*,*,#1915,.F.);
#2674=ORIENTED_EDGE('',*,*,#1928,.T.);
#2675=ORIENTED_EDGE('',*,*,#1929,.T.);
#2676=ORIENTED_EDGE('',*,*,#1930,.F.);
#2677=ORIENTED_EDGE('',*,*,#1931,.T.);
#2678=ORIENTED_EDGE('',*,*,#1932,.F.);
#2679=ORIENTED_EDGE('',*,*,#1933,.T.);
#2680=ORIENTED_EDGE('',*,*,#1934,.T.);
#2681=ORIENTED_EDGE('',*,*,#1909,.F.);
#2682=ORIENTED_EDGE('',*,*,#1935,.T.);
#2683=ORIENTED_EDGE('',*,*,#1936,.T.);
#2684=ORIENTED_EDGE('',*,*,#1937,.F.);
#2685=ORIENTED_EDGE('',*,*,#1938,.T.);
#2686=ORIENTED_EDGE('',*,*,#1939,.F.);
#2687=ORIENTED_EDGE('',*,*,#1940,.T.);
#2688=ORIENTED_EDGE('',*,*,#1941,.T.);
#2689=ORIENTED_EDGE('',*,*,#1911,.F.);
#2690=ORIENTED_EDGE('',*,*,#1942,.T.);
#2691=ORIENTED_EDGE('',*,*,#1943,.T.);
#2692=ORIENTED_EDGE('',*,*,#1944,.F.);
#2693=ORIENTED_EDGE('',*,*,#1945,.T.);
#2694=ORIENTED_EDGE('',*,*,#1946,.F.);
#2695=ORIENTED_EDGE('',*,*,#1947,.T.);
#2696=ORIENTED_EDGE('',*,*,#1948,.T.);
#2697=ORIENTED_EDGE('',*,*,#1904,.T.);
#2698=ORIENTED_EDGE('',*,*,#1949,.T.);
#2699=ORIENTED_EDGE('',*,*,#1950,.T.);
#2700=ORIENTED_EDGE('',*,*,#1951,.T.);
#2701=ORIENTED_EDGE('',*,*,#1950,.F.);
#2702=ORIENTED_EDGE('',*,*,#1887,.T.);
#2703=ORIENTED_EDGE('',*,*,#1888,.T.);
#2704=ORIENTED_EDGE('',*,*,#1951,.F.);
#2705=ORIENTED_EDGE('',*,*,#1895,.T.);
#2706=ORIENTED_EDGE('',*,*,#1905,.F.);
#2707=ORIENTED_EDGE('',*,*,#1902,.F.);
#2708=ORIENTED_EDGE('',*,*,#1900,.T.);
#2709=ORIENTED_EDGE('',*,*,#1890,.T.);
#2710=ORIENTED_EDGE('',*,*,#1918,.T.);
#2711=ORIENTED_EDGE('',*,*,#1952,.T.);
#2712=ORIENTED_EDGE('',*,*,#1953,.T.);
#2713=ORIENTED_EDGE('',*,*,#1952,.F.);
#2714=ORIENTED_EDGE('',*,*,#1953,.F.);
#2715=ORIENTED_EDGE('',*,*,#1949,.F.);
#2716=ORIENTED_EDGE('',*,*,#1945,.F.);
#2717=ORIENTED_EDGE('',*,*,#1954,.T.);
#2718=ORIENTED_EDGE('',*,*,#1955,.T.);
#2719=ORIENTED_EDGE('',*,*,#1956,.F.);
#2720=ORIENTED_EDGE('',*,*,#1944,.T.);
#2721=ORIENTED_EDGE('',*,*,#1957,.T.);
#2722=ORIENTED_EDGE('',*,*,#1958,.T.);
#2723=ORIENTED_EDGE('',*,*,#1954,.F.);
#2724=ORIENTED_EDGE('',*,*,#1943,.F.);
#2725=ORIENTED_EDGE('',*,*,#1959,.T.);
#2726=ORIENTED_EDGE('',*,*,#1960,.T.);
#2727=ORIENTED_EDGE('',*,*,#1957,.F.);
#2728=ORIENTED_EDGE('',*,*,#1942,.F.);
#2729=ORIENTED_EDGE('',*,*,#1910,.T.);
#2730=ORIENTED_EDGE('',*,*,#1924,.T.);
#2731=ORIENTED_EDGE('',*,*,#1961,.T.);
#2732=ORIENTED_EDGE('',*,*,#1959,.F.);
#2733=ORIENTED_EDGE('',*,*,#1948,.F.);
#2734=ORIENTED_EDGE('',*,*,#1962,.T.);
#2735=ORIENTED_EDGE('',*,*,#1963,.T.);
#2736=ORIENTED_EDGE('',*,*,#1922,.F.);
#2737=ORIENTED_EDGE('',*,*,#1916,.F.);
#2738=ORIENTED_EDGE('',*,*,#1947,.F.);
#2739=ORIENTED_EDGE('',*,*,#1964,.T.);
#2740=ORIENTED_EDGE('',*,*,#1965,.T.);
#2741=ORIENTED_EDGE('',*,*,#1962,.F.);
#2742=ORIENTED_EDGE('',*,*,#1946,.T.);
#2743=ORIENTED_EDGE('',*,*,#1956,.T.);
#2744=ORIENTED_EDGE('',*,*,#1966,.T.);
#2745=ORIENTED_EDGE('',*,*,#1964,.F.);
#2746=ORIENTED_EDGE('',*,*,#1966,.F.);
#2747=ORIENTED_EDGE('',*,*,#1955,.F.);
#2748=ORIENTED_EDGE('',*,*,#1958,.F.);
#2749=ORIENTED_EDGE('',*,*,#1960,.F.);
#2750=ORIENTED_EDGE('',*,*,#1961,.F.);
#2751=ORIENTED_EDGE('',*,*,#1923,.F.);
#2752=ORIENTED_EDGE('',*,*,#1963,.F.);
#2753=ORIENTED_EDGE('',*,*,#1965,.F.);
#2754=ORIENTED_EDGE('',*,*,#1938,.F.);
#2755=ORIENTED_EDGE('',*,*,#1967,.T.);
#2756=ORIENTED_EDGE('',*,*,#1968,.T.);
#2757=ORIENTED_EDGE('',*,*,#1969,.F.);
#2758=ORIENTED_EDGE('',*,*,#1937,.T.);
#2759=ORIENTED_EDGE('',*,*,#1970,.T.);
#2760=ORIENTED_EDGE('',*,*,#1971,.T.);
#2761=ORIENTED_EDGE('',*,*,#1967,.F.);
#2762=ORIENTED_EDGE('',*,*,#1936,.F.);
#2763=ORIENTED_EDGE('',*,*,#1972,.T.);
#2764=ORIENTED_EDGE('',*,*,#1973,.T.);
#2765=ORIENTED_EDGE('',*,*,#1970,.F.);
#2766=ORIENTED_EDGE('',*,*,#1935,.F.);
#2767=ORIENTED_EDGE('',*,*,#1908,.T.);
#2768=ORIENTED_EDGE('',*,*,#1927,.T.);
#2769=ORIENTED_EDGE('',*,*,#1974,.T.);
#2770=ORIENTED_EDGE('',*,*,#1972,.F.);
#2771=ORIENTED_EDGE('',*,*,#1941,.F.);
#2772=ORIENTED_EDGE('',*,*,#1975,.T.);
#2773=ORIENTED_EDGE('',*,*,#1976,.T.);
#2774=ORIENTED_EDGE('',*,*,#1925,.F.);
#2775=ORIENTED_EDGE('',*,*,#1912,.F.);
#2776=ORIENTED_EDGE('',*,*,#1940,.F.);
#2777=ORIENTED_EDGE('',*,*,#1977,.T.);
#2778=ORIENTED_EDGE('',*,*,#1978,.T.);
#2779=ORIENTED_EDGE('',*,*,#1975,.F.);
#2780=ORIENTED_EDGE('',*,*,#1939,.T.);
#2781=ORIENTED_EDGE('',*,*,#1969,.T.);
#2782=ORIENTED_EDGE('',*,*,#1979,.T.);
#2783=ORIENTED_EDGE('',*,*,#1977,.F.);
#2784=ORIENTED_EDGE('',*,*,#1979,.F.);
#2785=ORIENTED_EDGE('',*,*,#1968,.F.);
#2786=ORIENTED_EDGE('',*,*,#1971,.F.);
#2787=ORIENTED_EDGE('',*,*,#1973,.F.);
#2788=ORIENTED_EDGE('',*,*,#1974,.F.);
#2789=ORIENTED_EDGE('',*,*,#1926,.F.);
#2790=ORIENTED_EDGE('',*,*,#1976,.F.);
#2791=ORIENTED_EDGE('',*,*,#1978,.F.);
#2792=ORIENTED_EDGE('',*,*,#1931,.F.);
#2793=ORIENTED_EDGE('',*,*,#1980,.T.);
#2794=ORIENTED_EDGE('',*,*,#1981,.T.);
#2795=ORIENTED_EDGE('',*,*,#1982,.F.);
#2796=ORIENTED_EDGE('',*,*,#1930,.T.);
#2797=ORIENTED_EDGE('',*,*,#1983,.T.);
#2798=ORIENTED_EDGE('',*,*,#1984,.T.);
#2799=ORIENTED_EDGE('',*,*,#1980,.F.);
#2800=ORIENTED_EDGE('',*,*,#1929,.F.);
#2801=ORIENTED_EDGE('',*,*,#1985,.T.);
#2802=ORIENTED_EDGE('',*,*,#1986,.T.);
#2803=ORIENTED_EDGE('',*,*,#1983,.F.);
#2804=ORIENTED_EDGE('',*,*,#1928,.F.);
#2805=ORIENTED_EDGE('',*,*,#1914,.T.);
#2806=ORIENTED_EDGE('',*,*,#1987,.T.);
#2807=ORIENTED_EDGE('',*,*,#1988,.T.);
#2808=ORIENTED_EDGE('',*,*,#1985,.F.);
#2809=ORIENTED_EDGE('',*,*,#1921,.F.);
#2810=ORIENTED_EDGE('',*,*,#1989,.T.);
#2811=ORIENTED_EDGE('',*,*,#1990,.T.);
#2812=ORIENTED_EDGE('',*,*,#1987,.F.);
#2813=ORIENTED_EDGE('',*,*,#1934,.F.);
#2814=ORIENTED_EDGE('',*,*,#1991,.T.);
#2815=ORIENTED_EDGE('',*,*,#1992,.T.);
#2816=ORIENTED_EDGE('',*,*,#1989,.F.);
#2817=ORIENTED_EDGE('',*,*,#1906,.F.);
#2818=ORIENTED_EDGE('',*,*,#1933,.F.);
#2819=ORIENTED_EDGE('',*,*,#1993,.T.);
#2820=ORIENTED_EDGE('',*,*,#1994,.T.);
#2821=ORIENTED_EDGE('',*,*,#1991,.F.);
#2822=ORIENTED_EDGE('',*,*,#1932,.T.);
#2823=ORIENTED_EDGE('',*,*,#1982,.T.);
#2824=ORIENTED_EDGE('',*,*,#1995,.T.);
#2825=ORIENTED_EDGE('',*,*,#1993,.F.);
#2826=ORIENTED_EDGE('',*,*,#1995,.F.);
#2827=ORIENTED_EDGE('',*,*,#1981,.F.);
#2828=ORIENTED_EDGE('',*,*,#1984,.F.);
#2829=ORIENTED_EDGE('',*,*,#1986,.F.);
#2830=ORIENTED_EDGE('',*,*,#1988,.F.);
#2831=ORIENTED_EDGE('',*,*,#1990,.F.);
#2832=ORIENTED_EDGE('',*,*,#1992,.F.);
#2833=ORIENTED_EDGE('',*,*,#1994,.F.);
#3071=CYLINDRICAL_SURFACE('',#3567,1.);
#3072=CYLINDRICAL_SURFACE('',#3574,1.);
#3073=CYLINDRICAL_SURFACE('',#3576,5.);
#3074=CYLINDRICAL_SURFACE('',#3580,12.);
#3075=CYLINDRICAL_SURFACE('',#3583,12.);
#3076=CYLINDRICAL_SURFACE('',#3586,12.);
#3077=CYLINDRICAL_SURFACE('',#3594,12.);
#3078=CYLINDRICAL_SURFACE('',#3596,12.);
#3079=CYLINDRICAL_SURFACE('',#3608,7.);
#3080=CYLINDRICAL_SURFACE('',#3612,13.5);
#3081=CYLINDRICAL_SURFACE('',#3615,5.529);
#3082=CYLINDRICAL_SURFACE('',#3617,1.);
#3083=CYLINDRICAL_SURFACE('',#3621,1.);
#3084=CYLINDRICAL_SURFACE('',#3624,5.529);
#3085=CYLINDRICAL_SURFACE('',#3626,1.);
#3086=CYLINDRICAL_SURFACE('',#3630,1.);
#3087=CYLINDRICAL_SURFACE('',#3633,5.529);
#3088=CYLINDRICAL_SURFACE('',#3635,1.);
#3089=CYLINDRICAL_SURFACE('',#3638,12.);
#3090=CYLINDRICAL_SURFACE('',#3641,1.);
#3197=ADVANCED_FACE('',(#359),#3071,.F.);
#3198=ADVANCED_FACE('',(#360),#212,.F.);
#3199=ADVANCED_FACE('',(#361),#213,.F.);
#3200=ADVANCED_FACE('',(#362),#214,.T.);
#3201=ADVANCED_FACE('',(#363),#3072,.F.);
#3202=ADVANCED_FACE('',(#364),#215,.T.);
#3203=ADVANCED_FACE('',(#365),#3073,.F.);
#3204=ADVANCED_FACE('',(#366),#3074,.F.);
#3205=ADVANCED_FACE('',(#367),#3075,.F.);
#3206=ADVANCED_FACE('',(#368),#3076,.F.);
#3207=ADVANCED_FACE('',(#369,#90),#216,.T.);
#3208=ADVANCED_FACE('',(#370),#3077,.T.);
#3209=ADVANCED_FACE('',(#371),#3078,.T.);
#3210=ADVANCED_FACE('',(#372,#91),#217,.T.);
#3211=ADVANCED_FACE('',(#373,#92),#3079,.T.);
#3212=ADVANCED_FACE('',(#374,#93),#218,.F.);
#3213=ADVANCED_FACE('',(#375),#3080,.T.);
#3214=ADVANCED_FACE('',(#376,#94),#219,.F.);
#3215=ADVANCED_FACE('',(#377),#3081,.F.);
#3216=ADVANCED_FACE('',(#378),#3082,.T.);
#3217=ADVANCED_FACE('',(#379),#220,.F.);
#3218=ADVANCED_FACE('',(#380),#175,.F.);
#3219=ADVANCED_FACE('',(#381),#176,.F.);
#3220=ADVANCED_FACE('',(#382),#221,.F.);
#3221=ADVANCED_FACE('',(#383),#3083,.T.);
#3222=ADVANCED_FACE('',(#384),#222,.T.);
#3223=ADVANCED_FACE('',(#385),#3084,.F.);
#3224=ADVANCED_FACE('',(#386),#3085,.T.);
#3225=ADVANCED_FACE('',(#387),#223,.F.);
#3226=ADVANCED_FACE('',(#388),#177,.F.);
#3227=ADVANCED_FACE('',(#389),#178,.F.);
#3228=ADVANCED_FACE('',(#390),#224,.F.);
#3229=ADVANCED_FACE('',(#391),#3086,.T.);
#3230=ADVANCED_FACE('',(#392),#225,.T.);
#3231=ADVANCED_FACE('',(#393),#3087,.F.);
#3232=ADVANCED_FACE('',(#394),#3088,.T.);
#3233=ADVANCED_FACE('',(#395),#226,.F.);
#3234=ADVANCED_FACE('',(#396),#179,.F.);
#3235=ADVANCED_FACE('',(#397),#3089,.T.);
#3236=ADVANCED_FACE('',(#398),#180,.F.);
#3237=ADVANCED_FACE('',(#399),#227,.F.);
#3238=ADVANCED_FACE('',(#400),#3090,.T.);
#3239=ADVANCED_FACE('',(#401),#228,.T.);
#3290=CLOSED_SHELL('',(#3197,#3198,#3199,#3200,#3201,#3202,#3203,#3204,
#3205,#3206,#3207,#3208,#3209,#3210,#3211,#3212,#3213,#3214,#3215,#3216,
#3217,#3218,#3219,#3220,#3221,#3222,#3223,#3224,#3225,#3226,#3227,#3228,
#3229,#3230,#3231,#3232,#3233,#3234,#3235,#3236,#3237,#3238,#3239));
#3566=AXIS2_PLACEMENT_3D('',#9009,#4195,#4196);
#3567=AXIS2_PLACEMENT_3D('',#9010,#4197,#4198);
#3568=AXIS2_PLACEMENT_3D('',#9013,#4199,#4200);
#3569=AXIS2_PLACEMENT_3D('',#9014,#4201,#4202);
#3570=AXIS2_PLACEMENT_3D('',#9054,#4204,#4205);
#3571=AXIS2_PLACEMENT_3D('',#9060,#4209,#4210);
#3572=AXIS2_PLACEMENT_3D('',#9064,#4212,#4213);
#3573=AXIS2_PLACEMENT_3D('',#9066,#4215,#4216);
#3574=AXIS2_PLACEMENT_3D('',#9072,#4220,#4221);
#3575=AXIS2_PLACEMENT_3D('',#9093,#4223,#4224);
#3576=AXIS2_PLACEMENT_3D('',#9097,#4227,#4228);
#3577=AXIS2_PLACEMENT_3D('',#9099,#4229,#4230);
#3578=AXIS2_PLACEMENT_3D('',#9102,#4232,#4233);
#3579=AXIS2_PLACEMENT_3D('',#9103,#4234,#4235);
#3580=AXIS2_PLACEMENT_3D('',#9104,#4236,#4237);
#3581=AXIS2_PLACEMENT_3D('',#9109,#4239,#4240);
#3582=AXIS2_PLACEMENT_3D('',#9112,#4242,#4243);
#3583=AXIS2_PLACEMENT_3D('',#9113,#4244,#4245);
#3584=AXIS2_PLACEMENT_3D('',#9118,#4247,#4248);
#3585=AXIS2_PLACEMENT_3D('',#9121,#4250,#4251);
#3586=AXIS2_PLACEMENT_3D('',#9122,#4252,#4253);
#3587=AXIS2_PLACEMENT_3D('',#9127,#4255,#4256);
#3588=AXIS2_PLACEMENT_3D('',#9130,#4258,#4259);
#3589=AXIS2_PLACEMENT_3D('',#9131,#4260,#4261);
#3590=AXIS2_PLACEMENT_3D('',#9133,#4262,#4263);
#3591=AXIS2_PLACEMENT_3D('',#9134,#4264,#4265);
#3592=AXIS2_PLACEMENT_3D('',#9135,#4266,#4267);
#3593=AXIS2_PLACEMENT_3D('',#9136,#4268,#4269);
#3594=AXIS2_PLACEMENT_3D('',#9137,#4270,#4271);
#3595=AXIS2_PLACEMENT_3D('',#9141,#4273,#4274);
#3596=AXIS2_PLACEMENT_3D('',#9143,#4276,#4277);
#3597=AXIS2_PLACEMENT_3D('',#9147,#4279,#4280);
#3598=AXIS2_PLACEMENT_3D('',#9149,#4282,#4283);
#3599=AXIS2_PLACEMENT_3D('',#9164,#4285,#4286);
#3600=AXIS2_PLACEMENT_3D('',#9166,#4287,#4288);
#3601=AXIS2_PLACEMENT_3D('',#9168,#4289,#4290);
#3602=AXIS2_PLACEMENT_3D('',#9195,#4293,#4294);
#3603=AXIS2_PLACEMENT_3D('',#9197,#4295,#4296);
#3604=AXIS2_PLACEMENT_3D('',#9199,#4297,#4298);
#3605=AXIS2_PLACEMENT_3D('',#9226,#4301,#4302);
#3606=AXIS2_PLACEMENT_3D('',#9228,#4303,#4304);
#3607=AXIS2_PLACEMENT_3D('',#9230,#4305,#4306);
#3608=AXIS2_PLACEMENT_3D('',#9243,#4308,#4309);
#3609=AXIS2_PLACEMENT_3D('',#9245,#4310,#4311);
#3610=AXIS2_PLACEMENT_3D('',#9248,#4313,#4314);
#3611=AXIS2_PLACEMENT_3D('',#9249,#4315,#4316);
#3612=AXIS2_PLACEMENT_3D('',#9250,#4317,#4318);
#3613=AXIS2_PLACEMENT_3D('',#9253,#4320,#4321);
#3614=AXIS2_PLACEMENT_3D('',#9254,#4322,#4323);
#3615=AXIS2_PLACEMENT_3D('',#9255,#4324,#4325);
#3616=AXIS2_PLACEMENT_3D('',#9259,#4327,#4328);
#3617=AXIS2_PLACEMENT_3D('',#9261,#4330,#4331);
#3618=AXIS2_PLACEMENT_3D('',#9264,#4333,#4334);
#3619=AXIS2_PLACEMENT_3D('',#9265,#4335,#4336);
#3620=AXIS2_PLACEMENT_3D('',#9331,#4340,#4341);
#3621=AXIS2_PLACEMENT_3D('',#9335,#4344,#4345);
#3622=AXIS2_PLACEMENT_3D('',#9336,#4346,#4347);
#3623=AXIS2_PLACEMENT_3D('',#9337,#4348,#4349);
#3624=AXIS2_PLACEMENT_3D('',#9338,#4350,#4351);
#3625=AXIS2_PLACEMENT_3D('',#9342,#4353,#4354);
#3626=AXIS2_PLACEMENT_3D('',#9344,#4356,#4357);
#3627=AXIS2_PLACEMENT_3D('',#9347,#4359,#4360);
#3628=AXIS2_PLACEMENT_3D('',#9348,#4361,#4362);
#3629=AXIS2_PLACEMENT_3D('',#9414,#4366,#4367);
#3630=AXIS2_PLACEMENT_3D('',#9418,#4370,#4371);
#3631=AXIS2_PLACEMENT_3D('',#9419,#4372,#4373);
#3632=AXIS2_PLACEMENT_3D('',#9420,#4374,#4375);
#3633=AXIS2_PLACEMENT_3D('',#9421,#4376,#4377);
#3634=AXIS2_PLACEMENT_3D('',#9425,#4379,#4380);
#3635=AXIS2_PLACEMENT_3D('',#9427,#4382,#4383);
#3636=AXIS2_PLACEMENT_3D('',#9430,#4385,#4386);
#3637=AXIS2_PLACEMENT_3D('',#9431,#4387,#4388);
#3638=AXIS2_PLACEMENT_3D('',#9467,#4392,#4393);
#3639=AXIS2_PLACEMENT_3D('',#9470,#4395,#4396);
#3640=AXIS2_PLACEMENT_3D('',#9503,#4398,#4399);
#3641=AXIS2_PLACEMENT_3D('',#9507,#4402,#4403);
#3642=AXIS2_PLACEMENT_3D('',#9508,#4404,#4405);
#3643=AXIS2_PLACEMENT_3D('',#9509,#4406,#4407);
#4195=DIRECTION('axis',(0.,0.,1.));
#4196=DIRECTION('refdir',(1.,0.,0.));
#4197=DIRECTION('center_axis',(0.,-1.,0.));
#4198=DIRECTION('ref_axis',(1.,0.,0.));
#4199=DIRECTION('center_axis',(0.,-1.,0.));
#4200=DIRECTION('ref_axis',(1.,0.,0.));
#4201=DIRECTION('center_axis',(0.,-1.,0.));
#4202=DIRECTION('ref_axis',(1.,0.,0.));
#4203=DIRECTION('',(0.,-1.,0.));
#4204=DIRECTION('center_axis',(0.,-1.,0.));
#4205=DIRECTION('ref_axis',(1.,0.,0.));
#4206=DIRECTION('',(0.,0.,-1.));
#4207=DIRECTION('',(1.,0.,0.));
#4208=DIRECTION('',(0.,0.,1.));
#4209=DIRECTION('center_axis',(0.,-1.,0.));
#4210=DIRECTION('ref_axis',(1.,0.,0.));
#4211=DIRECTION('',(0.,0.,1.));
#4212=DIRECTION('center_axis',(0.,1.,0.));
#4213=DIRECTION('ref_axis',(1.,0.,0.));
#4214=DIRECTION('',(0.,0.,-1.));
#4215=DIRECTION('center_axis',(-1.,0.,0.));
#4216=DIRECTION('ref_axis',(0.,0.,-1.));
#4217=DIRECTION('',(0.,1.,0.));
#4218=DIRECTION('',(0.,-1.,0.));
#4219=DIRECTION('',(0.,0.,1.));
#4220=DIRECTION('center_axis',(0.,1.,0.));
#4221=DIRECTION('ref_axis',(1.,0.,0.));
#4222=DIRECTION('',(0.,-1.,0.));
#4223=DIRECTION('center_axis',(1.,0.,0.));
#4224=DIRECTION('ref_axis',(0.,0.,1.));
#4225=DIRECTION('',(0.,-1.,0.));
#4226=DIRECTION('',(0.,0.,-1.));
#4227=DIRECTION('center_axis',(0.,0.,1.));
#4228=DIRECTION('ref_axis',(0.5,-0.866025403784439,0.));
#4229=DIRECTION('center_axis',(0.,0.,-1.));
#4230=DIRECTION('ref_axis',(-0.5,0.866025403784439,0.));
#4231=DIRECTION('',(0.,0.,1.));
#4232=DIRECTION('center_axis',(0.,0.,-1.));
#4233=DIRECTION('ref_axis',(0.5,-0.866025403784439,0.));
#4234=DIRECTION('center_axis',(0.,0.,-1.));
#4235=DIRECTION('ref_axis',(-0.5,0.866025403784439,0.));
#4236=DIRECTION('center_axis',(0.,0.,-1.));
#4237=DIRECTION('ref_axis',(0.5,-0.866025403784439,0.));
#4238=DIRECTION('',(0.,0.,1.));
#4239=DIRECTION('center_axis',(0.,0.,1.));
#4240=DIRECTION('ref_axis',(0.5,-0.866025403784439,0.));
#4241=DIRECTION('',(0.,0.,1.));
#4242=DIRECTION('center_axis',(0.,0.,-1.));
#4243=DIRECTION('ref_axis',(0.5,-0.866025403784439,0.));
#4244=DIRECTION('center_axis',(0.,0.,-1.));
#4245=DIRECTION('ref_axis',(0.,1.,0.));
#4246=DIRECTION('',(0.,0.,1.));
#4247=DIRECTION('center_axis',(0.,0.,-1.));
#4248=DIRECTION('ref_axis',(0.5,-0.866025403784439,0.));
#4249=DIRECTION('',(0.,0.,1.));
#4250=DIRECTION('center_axis',(0.,0.,1.));
#4251=DIRECTION('ref_axis',(0.5,-0.866025403784439,0.));
#4252=DIRECTION('center_axis',(0.,0.,-1.));
#4253=DIRECTION('ref_axis',(0.5,-0.866025403784439,0.));
#4254=DIRECTION('',(0.,0.,1.));
#4255=DIRECTION('center_axis',(0.,0.,-1.));
#4256=DIRECTION('ref_axis',(0.5,-0.866025403784439,0.));
#4257=DIRECTION('',(0.,0.,1.));
#4258=DIRECTION('center_axis',(0.,0.,1.));
#4259=DIRECTION('ref_axis',(0.5,-0.866025403784439,0.));
#4260=DIRECTION('center_axis',(0.,0.,1.));
#4261=DIRECTION('ref_axis',(0.5,-0.866025403784439,0.));
#4262=DIRECTION('center_axis',(0.,0.,-1.));
#4263=DIRECTION('ref_axis',(0.5,-0.866025403784439,0.));
#4264=DIRECTION('center_axis',(0.,0.,-1.));
#4265=DIRECTION('ref_axis',(0.5,-0.866025403784439,0.));
#4266=DIRECTION('center_axis',(0.,0.,-1.));
#4267=DIRECTION('ref_axis',(0.5,-0.866025403784439,0.));
#4268=DIRECTION('center_axis',(0.,0.,-1.));
#4269=DIRECTION('ref_axis',(0.5,-0.866025403784439,0.));
#4270=DIRECTION('center_axis',(0.,0.,-1.));
#4271=DIRECTION('ref_axis',(0.5,-0.866025403784439,0.));
#4272=DIRECTION('',(0.,0.,1.));
#4273=DIRECTION('center_axis',(0.,0.,-1.));
#4274=DIRECTION('ref_axis',(0.5,-0.866025403784439,0.));
#4275=DIRECTION('',(0.,0.,1.));
#4276=DIRECTION('center_axis',(0.,0.,-1.));
#4277=DIRECTION('ref_axis',(0.5,-0.866025403784439,0.));
#4278=DIRECTION('',(0.,0.,1.));
#4279=DIRECTION('center_axis',(0.,0.,-1.));
#4280=DIRECTION('ref_axis',(0.5,-0.866025403784439,0.));
#4281=DIRECTION('',(0.,0.,1.));
#4282=DIRECTION('center_axis',(0.,0.,1.));
#4283=DIRECTION('ref_axis',(0.5,-0.866025403784439,0.));
#4284=DIRECTION('',(0.244394302218901,0.969675938158175,0.));
#4285=DIRECTION('center_axis',(0.,0.,1.));
#4286=DIRECTION('ref_axis',(0.092992392522802,0.995666819238687,0.));
#4287=DIRECTION('center_axis',(0.,0.,1.));
#4288=DIRECTION('ref_axis',(-0.0929923925228033,-0.995666819238687,0.));
#4289=DIRECTION('center_axis',(0.,0.,1.));
#4290=DIRECTION('ref_axis',(0.969675938158175,0.244394302218901,0.));
#4291=DIRECTION('',(0.244394302218901,-0.969675938158175,0.));
#4292=DIRECTION('',(-0.961961146992938,-0.273186294817348,0.));
#4293=DIRECTION('center_axis',(0.,0.,1.));
#4294=DIRECTION('ref_axis',(-0.908768955427354,-0.417299635335902,0.));
#4295=DIRECTION('center_axis',(0.,0.,1.));
#4296=DIRECTION('ref_axis',(0.908768955427354,0.417299635335902,0.));
#4297=DIRECTION('center_axis',(0.,0.,1.));
#4298=DIRECTION('ref_axis',(-0.696489643340827,0.717566844774037,0.));
#4299=DIRECTION('',(0.717566844774038,0.696489643340827,0.));
#4300=DIRECTION('',(0.717566844774037,-0.696489643340827,0.));
#4301=DIRECTION('center_axis',(0.,0.,1.));
#4302=DIRECTION('ref_axis',(0.81577656290455,-0.578367183902785,0.));
#4303=DIRECTION('center_axis',(0.,0.,1.));
#4304=DIRECTION('ref_axis',(-0.815776562904551,0.578367183902785,0.));
#4305=DIRECTION('center_axis',(0.,0.,1.));
#4306=DIRECTION('ref_axis',(-0.273186294817348,-0.961961146992938,0.));
#4307=DIRECTION('',(-0.961961146992938,0.273186294817348,0.));
#4308=DIRECTION('center_axis',(0.,0.,1.));
#4309=DIRECTION('ref_axis',(-0.5,0.866025403784439,0.));
#4310=DIRECTION('center_axis',(0.,0.,1.));
#4311=DIRECTION('ref_axis',(-0.5,0.866025403784439,0.));
#4312=DIRECTION('',(0.,0.,-1.));
#4313=DIRECTION('center_axis',(0.,0.,1.));
#4314=DIRECTION('ref_axis',(-0.5,0.866025403784439,0.));
#4315=DIRECTION('center_axis',(0.,0.,1.));
#4316=DIRECTION('ref_axis',(-0.5,0.866025403784439,0.));
#4317=DIRECTION('center_axis',(0.,0.,1.));
#4318=DIRECTION('ref_axis',(0.5,-0.866025403784439,0.));
#4319=DIRECTION('',(0.,0.,-1.));
#4320=DIRECTION('center_axis',(0.,0.,1.));
#4321=DIRECTION('ref_axis',(0.5,-0.866025403784439,0.));
#4322=DIRECTION('center_axis',(0.,0.,1.));
#4323=DIRECTION('ref_axis',(0.5,-0.866025403784439,0.));
#4324=DIRECTION('center_axis',(0.,0.,-1.));
#4325=DIRECTION('ref_axis',(-0.815776562904551,0.578367183902785,0.));
#4326=DIRECTION('',(0.,0.,1.));
#4327=DIRECTION('center_axis',(0.,0.,1.));
#4328=DIRECTION('ref_axis',(-0.815776562904551,0.578367183902785,0.));
#4329=DIRECTION('',(0.,0.,1.));
#4330=DIRECTION('center_axis',(0.,0.,-1.));
#4331=DIRECTION('ref_axis',(0.81577656290455,-0.578367183902785,0.));
#4332=DIRECTION('',(0.,0.,1.));
#4333=DIRECTION('center_axis',(0.,0.,-1.));
#4334=DIRECTION('ref_axis',(0.81577656290455,-0.578367183902785,0.));
#4335=DIRECTION('center_axis',(-0.696489643340827,-0.717566844774037,0.));
#4336=DIRECTION('ref_axis',(0.717566844774037,-0.696489643340827,0.));
#4337=DIRECTION('',(0.,0.,1.));
#4338=DIRECTION('',(0.717566844774037,-0.696489643340827,0.));
#4339=DIRECTION('',(0.,0.,1.));
#4340=DIRECTION('center_axis',(0.273186294817348,0.961961146992938,0.));
#4341=DIRECTION('ref_axis',(-0.961961146992938,0.273186294817348,0.));
#4342=DIRECTION('',(0.,0.,1.));
#4343=DIRECTION('',(-0.961961146992938,0.273186294817348,0.));
#4344=DIRECTION('center_axis',(0.,0.,-1.));
#4345=DIRECTION('ref_axis',(-0.273186294817348,-0.961961146992938,0.));
#4346=DIRECTION('center_axis',(0.,0.,-1.));
#4347=DIRECTION('ref_axis',(-0.273186294817348,-0.961961146992938,0.));
#4348=DIRECTION('center_axis',(0.,0.,1.));
#4349=DIRECTION('ref_axis',(0.5,-0.866025403784439,0.));
#4350=DIRECTION('center_axis',(0.,0.,-1.));
#4351=DIRECTION('ref_axis',(0.908768955427354,0.417299635335902,0.));
#4352=DIRECTION('',(0.,0.,1.));
#4353=DIRECTION('center_axis',(0.,0.,1.));
#4354=DIRECTION('ref_axis',(0.908768955427354,0.417299635335902,0.));
#4355=DIRECTION('',(0.,0.,1.));
#4356=DIRECTION('center_axis',(0.,0.,-1.));
#4357=DIRECTION('ref_axis',(-0.908768955427354,-0.417299635335902,0.));
#4358=DIRECTION('',(0.,0.,1.));
#4359=DIRECTION('center_axis',(0.,0.,-1.));
#4360=DIRECTION('ref_axis',(-0.908768955427354,-0.417299635335902,0.));
#4361=DIRECTION('center_axis',(-0.273186294817348,0.961961146992938,0.));
#4362=DIRECTION('ref_axis',(-0.961961146992938,-0.273186294817348,0.));
#4363=DIRECTION('',(0.,0.,1.));
#4364=DIRECTION('',(-0.961961146992938,-0.273186294817348,0.));
#4365=DIRECTION('',(0.,0.,1.));
#4366=DIRECTION('center_axis',(0.696489643340827,-0.717566844774038,0.));
#4367=DIRECTION('ref_axis',(0.717566844774038,0.696489643340827,0.));
#4368=DIRECTION('',(0.,0.,1.));
#4369=DIRECTION('',(0.717566844774038,0.696489643340827,0.));
#4370=DIRECTION('center_axis',(0.,0.,-1.));
#4371=DIRECTION('ref_axis',(-0.696489643340827,0.717566844774037,0.));
#4372=DIRECTION('center_axis',(0.,0.,-1.));
#4373=DIRECTION('ref_axis',(-0.696489643340827,0.717566844774037,0.));
#4374=DIRECTION('center_axis',(0.,0.,1.));
#4375=DIRECTION('ref_axis',(0.5,-0.866025403784439,0.));
#4376=DIRECTION('center_axis',(0.,0.,-1.));
#4377=DIRECTION('ref_axis',(-0.0929923925228033,-0.995666819238687,0.));
#4378=DIRECTION('',(0.,0.,1.));
#4379=DIRECTION('center_axis',(0.,0.,1.));
#4380=DIRECTION('ref_axis',(-0.0929923925228033,-0.995666819238687,0.));
#4381=DIRECTION('',(0.,0.,1.));
#4382=DIRECTION('center_axis',(0.,0.,-1.));
#4383=DIRECTION('ref_axis',(0.092992392522802,0.995666819238687,0.));
#4384=DIRECTION('',(0.,0.,1.));
#4385=DIRECTION('center_axis',(0.,0.,-1.));
#4386=DIRECTION('ref_axis',(0.092992392522802,0.995666819238687,0.));
#4387=DIRECTION('center_axis',(0.969675938158175,-0.244394302218901,0.));
#4388=DIRECTION('ref_axis',(0.244394302218901,0.969675938158175,0.));
#4389=DIRECTION('',(0.,0.,1.));
#4390=DIRECTION('',(0.244394302218901,0.969675938158175,0.));
#4391=DIRECTION('',(0.,0.,1.));
#4392=DIRECTION('center_axis',(0.,0.,-1.));
#4393=DIRECTION('ref_axis',(0.5,-0.866025403784439,0.));
#4394=DIRECTION('',(0.,0.,1.));
#4395=DIRECTION('center_axis',(0.,0.,-1.));
#4396=DIRECTION('ref_axis',(0.5,-0.866025403784439,0.));
#4397=DIRECTION('',(0.,0.,1.));
#4398=DIRECTION('center_axis',(-0.969675938158175,-0.244394302218901,0.));
#4399=DIRECTION('ref_axis',(0.244394302218901,-0.969675938158175,0.));
#4400=DIRECTION('',(0.,0.,1.));
#4401=DIRECTION('',(0.244394302218901,-0.969675938158175,0.));
#4402=DIRECTION('center_axis',(0.,0.,-1.));
#4403=DIRECTION('ref_axis',(0.969675938158175,0.244394302218901,0.));
#4404=DIRECTION('center_axis',(0.,0.,-1.));
#4405=DIRECTION('ref_axis',(0.969675938158175,0.244394302218901,0.));
#4406=DIRECTION('center_axis',(0.,0.,1.));
#4407=DIRECTION('ref_axis',(0.5,-0.866025403784439,0.));
#9009=CARTESIAN_POINT('',(0.,0.,0.));
#9010=CARTESIAN_POINT('Origin',(0.,-6.,-9.));
#9011=CARTESIAN_POINT('',(1.,-6.,-9.));
#9012=CARTESIAN_POINT('',(-1.,-6.,-9.));
#9013=CARTESIAN_POINT('Origin',(0.,-6.,-9.));
#9014=CARTESIAN_POINT('Origin',(0.,-6.,-9.));
#9015=CARTESIAN_POINT('',(-1.,-6.92820323027551,-9.));
#9016=CARTESIAN_POINT('',(-1.,-6.,-9.));
#9017=CARTESIAN_POINT('',(1.,-6.92820323027551,-9.));
#9018=CARTESIAN_POINT('Ctrl Pts',(1.,-6.92820323027551,-9.));
#9019=CARTESIAN_POINT('Ctrl Pts',(1.,-6.92820323027551,-9.12574806852124));
#9020=CARTESIAN_POINT('Ctrl Pts',(0.974833943897391,-6.93198034025289,-9.25975855807223));
#9021=CARTESIAN_POINT('Ctrl Pts',(0.872727208600932,-6.94557411965751,-9.50608593513711));
#9022=CARTESIAN_POINT('Ctrl Pts',(0.795795807000654,-6.95518913236708,-9.61841775537244));
#9023=CARTESIAN_POINT('Ctrl Pts',(0.618419025069236,-6.97319901589886,-9.79579453730386));
#9024=CARTESIAN_POINT('Ctrl Pts',(0.506086655807109,-6.98277103675548,-9.87272693470229));
#9025=CARTESIAN_POINT('Ctrl Pts',(0.259757407800085,-6.99626622874452,-9.97483439587313));
#9026=CARTESIAN_POINT('Ctrl Pts',(0.125746268276869,-7.,-10.));
#9027=CARTESIAN_POINT('Ctrl Pts',(-0.125746268276869,-7.,-10.));
#9028=CARTESIAN_POINT('Ctrl Pts',(-0.259757407800085,-6.99626622874452,
-9.97483439587313));
#9029=CARTESIAN_POINT('Ctrl Pts',(-0.506086655807109,-6.98277103675548,
-9.87272693470229));
#9030=CARTESIAN_POINT('Ctrl Pts',(-0.618419025069236,-6.97319901589886,
-9.79579453730386));
#9031=CARTESIAN_POINT('Ctrl Pts',(-0.795795807000653,-6.95518913236708,
-9.61841775537244));
#9032=CARTESIAN_POINT('Ctrl Pts',(-0.872727208600932,-6.94557411965751,
-9.50608593513711));
#9033=CARTESIAN_POINT('Ctrl Pts',(-0.974833943897391,-6.93198034025289,
-9.25975855807223));
#9034=CARTESIAN_POINT('Ctrl Pts',(-1.,-6.92820323027551,-9.12574806852124));
#9035=CARTESIAN_POINT('Ctrl Pts',(-1.,-6.92820323027551,-9.));
#9036=CARTESIAN_POINT('Ctrl Pts',(-1.,-6.92820323027551,-9.));
#9037=CARTESIAN_POINT('Ctrl Pts',(-1.,-6.92820323027551,-8.87425193147876));
#9038=CARTESIAN_POINT('Ctrl Pts',(-0.974833943897391,-6.93198034025289,
-8.74024144192777));
#9039=CARTESIAN_POINT('Ctrl Pts',(-0.872727208600932,-6.94557411965751,
-8.49391406486289));
#9040=CARTESIAN_POINT('Ctrl Pts',(-0.795795807000653,-6.95518913236708,
-8.38158224462756));
#9041=CARTESIAN_POINT('Ctrl Pts',(-0.618419025069235,-6.97319901589886,
-8.20420546269614));
#9042=CARTESIAN_POINT('Ctrl Pts',(-0.506086655807108,-6.98277103675548,
-8.12727306529771));
#9043=CARTESIAN_POINT('Ctrl Pts',(-0.259757407800085,-6.99626622874452,
-8.02516560412687));
#9044=CARTESIAN_POINT('Ctrl Pts',(-0.125746268276869,-7.,-8.));
#9045=CARTESIAN_POINT('Ctrl Pts',(0.125746268276869,-7.,-8.));
#9046=CARTESIAN_POINT('Ctrl Pts',(0.259757407800085,-6.99626622874452,-8.02516560412687));
#9047=CARTESIAN_POINT('Ctrl Pts',(0.506086655807109,-6.98277103675548,-8.12727306529771));
#9048=CARTESIAN_POINT('Ctrl Pts',(0.618419025069235,-6.97319901589886,-8.20420546269614));
#9049=CARTESIAN_POINT('Ctrl Pts',(0.795795807000653,-6.95518913236708,-8.38158224462756));
#9050=CARTESIAN_POINT('Ctrl Pts',(0.872727208600931,-6.94557411965751,-8.49391406486289));
#9051=CARTESIAN_POINT('Ctrl Pts',(0.974833943897391,-6.93198034025289,-8.74024144192777));
#9052=CARTESIAN_POINT('Ctrl Pts',(1.,-6.92820323027551,-8.87425193147876));
#9053=CARTESIAN_POINT('Ctrl Pts',(1.,-6.92820323027551,-9.));
#9054=CARTESIAN_POINT('Origin',(0.,-6.,-10.5));
#9055=CARTESIAN_POINT('',(1.,-6.,-12.));
#9056=CARTESIAN_POINT('',(1.,-6.,-14.5));
#9057=CARTESIAN_POINT('',(-1.,-6.,-12.));
#9058=CARTESIAN_POINT('',(0.,-6.,-12.));
#9059=CARTESIAN_POINT('',(-1.,-6.,-6.5));
#9060=CARTESIAN_POINT('Origin',(0.,-6.,-10.5));
#9061=CARTESIAN_POINT('',(-1.,-6.,-6.5));
#9062=CARTESIAN_POINT('',(-1.,-6.,-6.5));
#9063=CARTESIAN_POINT('',(1.,-6.,-6.5));
#9064=CARTESIAN_POINT('Origin',(0.,-6.,-6.5));
#9065=CARTESIAN_POINT('',(1.,-6.,-14.5));
#9066=CARTESIAN_POINT('Origin',(1.,0.,-6.5));
#9067=CARTESIAN_POINT('',(1.,-4.89897948556636,-12.));
#9068=CARTESIAN_POINT('',(1.,0.,-12.));
#9069=CARTESIAN_POINT('',(1.,-4.89897948556636,-6.5));
#9070=CARTESIAN_POINT('',(1.,0.,-6.5));
#9071=CARTESIAN_POINT('',(1.,-4.89897948556636,-5.));
#9072=CARTESIAN_POINT('Origin',(0.,0.,-6.5));
#9073=CARTESIAN_POINT('',(-1.,-4.89897948556636,-6.5));
#9074=CARTESIAN_POINT('Ctrl Pts',(1.,-4.89897948556636,-6.5));
#9075=CARTESIAN_POINT('Ctrl Pts',(1.,-4.89897948556636,-6.3740682480366));
#9076=CARTESIAN_POINT('Ctrl Pts',(0.974762796248615,-4.90433876618447,-6.23998222283811));
#9077=CARTESIAN_POINT('Ctrl Pts',(0.872605417648384,-4.92354150792771,-5.99370799496995));
#9078=CARTESIAN_POINT('Ctrl Pts',(0.795703102192088,-4.93709085101933,-5.88148953981899));
#9079=CARTESIAN_POINT('Ctrl Pts',(0.618515424645094,-4.96240337638318,-5.704301862272));
#9080=CARTESIAN_POINT('Ctrl Pts',(0.506294861197626,-4.97583347151864,-5.62739565845524));
#9081=CARTESIAN_POINT('Ctrl Pts',(0.260013306081865,-4.99476188647081,-5.52523545776417));
#9082=CARTESIAN_POINT('Ctrl Pts',(0.125924695421399,-5.,-5.5));
#9083=CARTESIAN_POINT('Ctrl Pts',(-0.1259246954214,-5.,-5.5));
#9084=CARTESIAN_POINT('Ctrl Pts',(-0.260013306081865,-4.99476188647081,
-5.52523545776417));
#9085=CARTESIAN_POINT('Ctrl Pts',(-0.506294861197626,-4.97583347151864,
-5.62739565845524));
#9086=CARTESIAN_POINT('Ctrl Pts',(-0.618515424645094,-4.96240337638318,
-5.704301862272));
#9087=CARTESIAN_POINT('Ctrl Pts',(-0.795703102192089,-4.93709085101933,
-5.88148953981899));
#9088=CARTESIAN_POINT('Ctrl Pts',(-0.872605417648382,-4.92354150792771,
-5.99370799496995));
#9089=CARTESIAN_POINT('Ctrl Pts',(-0.974762796248614,-4.90433876618447,
-6.23998222283811));
#9090=CARTESIAN_POINT('Ctrl Pts',(-1.,-4.89897948556636,-6.3740682480366));
#9091=CARTESIAN_POINT('Ctrl Pts',(-1.,-4.89897948556636,-6.5));
#9092=CARTESIAN_POINT('',(-1.,0.,-6.5));
#9093=CARTESIAN_POINT('Origin',(-1.,0.,-14.5));
#9094=CARTESIAN_POINT('',(-1.,-4.89897948556636,-12.));
#9095=CARTESIAN_POINT('',(-1.,0.,-12.));
#9096=CARTESIAN_POINT('',(-1.,-4.89897948556636,-5.));
#9097=CARTESIAN_POINT('Origin',(0.,0.,-5.));
#9098=CARTESIAN_POINT('',(-2.5,4.33012701892219,-12.));
#9099=CARTESIAN_POINT('Origin',(0.,0.,-12.));
#9100=CARTESIAN_POINT('',(-2.5,4.33012701892219,-5.));
#9101=CARTESIAN_POINT('',(-2.5,4.33012701892219,-5.));
#9102=CARTESIAN_POINT('Origin',(0.,0.,-5.));
#9103=CARTESIAN_POINT('Origin',(0.,0.,-12.));
#9104=CARTESIAN_POINT('Origin',(0.,0.,-5.));
#9105=CARTESIAN_POINT('',(5.37912937500617,-10.726833976852,-5.));
#9106=CARTESIAN_POINT('',(5.37912937500617,-10.726833976852,-0.2));
#9107=CARTESIAN_POINT('',(5.37912937500617,-10.726833976852,-5.));
#9108=CARTESIAN_POINT('',(11.9792754136349,0.704954299427522,-0.2));
#9109=CARTESIAN_POINT('Origin',(0.,0.,-0.2));
#9110=CARTESIAN_POINT('',(11.9792754136349,0.704954299427527,-5.));
#9111=CARTESIAN_POINT('',(11.9792754136349,0.704954299427527,-5.));
#9112=CARTESIAN_POINT('Origin',(0.,0.,-5.));
#9113=CARTESIAN_POINT('Origin',(0.,0.,-5.));
#9114=CARTESIAN_POINT('',(-6.60014603862877,10.0218796774244,-5.));
#9115=CARTESIAN_POINT('',(-6.60014603862875,10.0218796774245,-0.2));
#9116=CARTESIAN_POINT('',(-6.60014603862877,10.0218796774244,-5.));
#9117=CARTESIAN_POINT('',(6.60014603862878,10.0218796774244,-5.));
#9118=CARTESIAN_POINT('Origin',(0.,0.,-5.));
#9119=CARTESIAN_POINT('',(6.60014603862878,10.0218796774244,-0.2));
#9120=CARTESIAN_POINT('',(6.60014603862878,10.0218796774244,-5.));
#9121=CARTESIAN_POINT('Origin',(0.,0.,-0.2));
#9122=CARTESIAN_POINT('Origin',(0.,0.,-5.));
#9123=CARTESIAN_POINT('',(-5.37912937500618,-10.726833976852,-5.));
#9124=CARTESIAN_POINT('',(-5.37912937500617,-10.726833976852,-0.2));
#9125=CARTESIAN_POINT('',(-5.37912937500618,-10.726833976852,-5.));
#9126=CARTESIAN_POINT('',(-11.9792754136349,0.704954299427533,-5.));
#9127=CARTESIAN_POINT('Origin',(0.,0.,-5.));
#9128=CARTESIAN_POINT('',(-11.9792754136349,0.704954299427533,-0.2));
#9129=CARTESIAN_POINT('',(-11.9792754136349,0.704954299427533,-5.));
#9130=CARTESIAN_POINT('Origin',(0.,0.,-0.2));
#9131=CARTESIAN_POINT('Origin',(0.,0.,-0.2));
#9132=CARTESIAN_POINT('',(-6.75,11.6913429510899,-0.2));
#9133=CARTESIAN_POINT('Origin',(0.,0.,-0.2));
#9134=CARTESIAN_POINT('Origin',(0.,0.,-0.2));
#9135=CARTESIAN_POINT('Origin',(0.,0.,-0.2));
#9136=CARTESIAN_POINT('Origin',(0.,0.,-0.2));
#9137=CARTESIAN_POINT('Origin',(0.,0.,-5.));
#9138=CARTESIAN_POINT('',(-11.9792754136349,0.704954299427533,1.5));
#9139=CARTESIAN_POINT('',(-11.9792754136349,0.704954299427533,-5.));
#9140=CARTESIAN_POINT('',(-6.60014603862877,10.0218796774244,1.5));
#9141=CARTESIAN_POINT('Origin',(0.,0.,1.5));
#9142=CARTESIAN_POINT('',(-6.60014603862877,10.0218796774244,-5.));
#9143=CARTESIAN_POINT('Origin',(0.,0.,-5.));
#9144=CARTESIAN_POINT('',(6.60014603862878,10.0218796774244,1.5));
#9145=CARTESIAN_POINT('',(6.60014603862878,10.0218796774244,-5.));
#9146=CARTESIAN_POINT('',(11.9792754136349,0.704954299427527,1.5));
#9147=CARTESIAN_POINT('Origin',(0.,0.,1.5));
#9148=CARTESIAN_POINT('',(11.9792754136349,0.704954299427527,-5.));
#9149=CARTESIAN_POINT('Origin',(0.,0.,-5.));
#9150=CARTESIAN_POINT('',(-2.06689970121501,-8.20077591276801,-5.));
#9151=CARTESIAN_POINT('Ctrl Pts',(-5.37912937500618,-10.726833976852,-5.));
#9152=CARTESIAN_POINT('Ctrl Pts',(-4.89017555905846,-10.5662385502925,-5.));
#9153=CARTESIAN_POINT('Ctrl Pts',(-4.41477448471897,-10.3612266948947,-5.));
#9154=CARTESIAN_POINT('Ctrl Pts',(-3.39025891465935,-9.77652560339542,-5.));
#9155=CARTESIAN_POINT('Ctrl Pts',(-3.02359566682149,-9.45605983842045,-5.));
#9156=CARTESIAN_POINT('Ctrl Pts',(-2.45567687261362,-8.90815881193254,-5.));
#9157=CARTESIAN_POINT('Ctrl Pts',(-2.27521579794306,-8.62451189270596,-5.));
#9158=CARTESIAN_POINT('Ctrl Pts',(-2.11932285414849,-8.34658168851868,-5.));
#9159=CARTESIAN_POINT('Ctrl Pts',(-2.0864345345459,-8.27828368469604,-5.));
#9160=CARTESIAN_POINT('Ctrl Pts',(-2.06689970121501,-8.20077591276801,-5.));
#9161=CARTESIAN_POINT('',(-1.57682326893956,-6.25631436059049,-5.));
#9162=CARTESIAN_POINT('',(-2.06689970121501,-8.20077591276801,-5.));
#9163=CARTESIAN_POINT('',(-0.51415493825858,-5.5050418435707,-5.));
#9164=CARTESIAN_POINT('Origin',(-0.607147330781382,-6.50070866280939,-5.));
#9165=CARTESIAN_POINT('',(0.514154938258578,-5.5050418435707,-5.));
#9166=CARTESIAN_POINT('Origin',(0.,0.,-5.));
#9167=CARTESIAN_POINT('',(1.57682326893955,-6.25631436059049,-5.));
#9168=CARTESIAN_POINT('Origin',(0.607147330781379,-6.50070866280939,-5.));
#9169=CARTESIAN_POINT('',(2.066899701215,-8.20077591276801,-5.));
#9170=CARTESIAN_POINT('',(1.57682326893955,-6.25631436059049,-5.));
#9171=CARTESIAN_POINT('Ctrl Pts',(2.066899701215,-8.20077591276801,-5.));
#9172=CARTESIAN_POINT('Ctrl Pts',(2.105832509837,-8.35524844908701,-5.));
#9173=CARTESIAN_POINT('Ctrl Pts',(2.19795327161749,-8.49250584591635,-5.));
#9174=CARTESIAN_POINT('Ctrl Pts',(2.30936577701074,-8.66518242906081,-5.));
#9175=CARTESIAN_POINT('Ctrl Pts',(2.40685301751416,-8.81420265426653,-5.));
#9176=CARTESIAN_POINT('Ctrl Pts',(2.70971882824218,-9.15550613959305,-5.));
#9177=CARTESIAN_POINT('Ctrl Pts',(2.95666208631803,-9.41660130067616,-5.));
#9178=CARTESIAN_POINT('Ctrl Pts',(3.90440084969946,-10.1119009779187,-5.));
#9179=CARTESIAN_POINT('Ctrl Pts',(4.57844358216429,-10.4638511096618,-5.));
#9180=CARTESIAN_POINT('Ctrl Pts',(5.37912937500617,-10.726833976852,-5.));
#9181=CARTESIAN_POINT('',(8.13553012180811,2.31040030805735,-5.));
#9182=CARTESIAN_POINT('Ctrl Pts',(11.9792754136349,0.704954299427528,-5.));
#9183=CARTESIAN_POINT('Ctrl Pts',(11.5957187866216,1.04810301195305,-5.));
#9184=CARTESIAN_POINT('Ctrl Pts',(11.1804727745766,1.35730649166136,-5.));
#9185=CARTESIAN_POINT('Ctrl Pts',(10.1618489906858,1.95221245615685,-5.));
#9186=CARTESIAN_POINT('Ctrl Pts',(9.70098587343182,2.10951926090029,-5.));
#9187=CARTESIAN_POINT('Ctrl Pts',(8.94253026837877,2.32740085079939,-5.));
#9188=CARTESIAN_POINT('Ctrl Pts',(8.60665429329664,2.34186126624275,-5.));
#9189=CARTESIAN_POINT('Ctrl Pts',(8.28801320409168,2.33790341374574,-5.));
#9190=CARTESIAN_POINT('Ctrl Pts',(8.21242123795344,2.33223653209797,-5.));
#9191=CARTESIAN_POINT('Ctrl Pts',(8.13553012180811,2.31040030805735,-5.));
#9192=CARTESIAN_POINT('',(6.20653880480254,1.76258817211517,-5.));
#9193=CARTESIAN_POINT('',(8.13553012180811,2.31040030805735,-5.));
#9194=CARTESIAN_POINT('',(5.02458355455784,2.3072496837722,-5.));
#9195=CARTESIAN_POINT('Origin',(5.93335250998519,2.72454931910811,-5.));
#9196=CARTESIAN_POINT('',(4.51042861629926,3.1977921597985,-5.));
#9197=CARTESIAN_POINT('Origin',(0.,0.,-5.));
#9198=CARTESIAN_POINT('',(4.62971553586298,4.49372618847532,-5.));
#9199=CARTESIAN_POINT('Origin',(5.32620517920381,3.77615934370128,-5.));
#9200=CARTESIAN_POINT('',(6.06863042059311,5.89037560471066,-5.));
#9201=CARTESIAN_POINT('',(4.62971553586298,4.49372618847532,-5.));
#9202=CARTESIAN_POINT('Ctrl Pts',(6.06863042059311,5.89037560471066,-5.));
#9203=CARTESIAN_POINT('Ctrl Pts',(6.18294115692139,6.00132867417748,-5.));
#9204=CARTESIAN_POINT('Ctrl Pts',(6.25574916854267,6.14973629251004,-5.));
#9205=CARTESIAN_POINT('Ctrl Pts',(6.34958522348502,6.3325606440466,-5.));
#9206=CARTESIAN_POINT('Ctrl Pts',(6.4298969039412,6.49149718347355,-5.));
#9207=CARTESIAN_POINT('Ctrl Pts',(6.57404148726847,6.92443841215994,-5.));
#9208=CARTESIAN_POINT('Ctrl Pts',(6.67668490053567,7.26884512749145,-5.));
#9209=CARTESIAN_POINT('Ctrl Pts',(6.80496270256398,8.43726081120601,-5.));
#9210=CARTESIAN_POINT('Ctrl Pts',(6.77273909133898,9.19697400660618,-5.));
#9211=CARTESIAN_POINT('Ctrl Pts',(6.60014603862878,10.0218796774244,-5.));
#9212=CARTESIAN_POINT('',(-6.06863042059311,5.89037560471066,-5.));
#9213=CARTESIAN_POINT('Ctrl Pts',(-6.60014603862877,10.0218796774244,-5.));
#9214=CARTESIAN_POINT('Ctrl Pts',(-6.70554322746249,9.51813553829505,-5.));
#9215=CARTESIAN_POINT('Ctrl Pts',(-6.76569828978797,9.00392020322571,-5.));
#9216=CARTESIAN_POINT('Ctrl Pts',(-6.77159007596056,7.82431314720816,-5.));
#9217=CARTESIAN_POINT('Ctrl Pts',(-6.67739020638207,7.34654057751468,-5.));
#9218=CARTESIAN_POINT('Ctrl Pts',(-6.48685339577862,6.58075796115043,-5.));
#9219=CARTESIAN_POINT('Ctrl Pts',(-6.33143849535641,6.28265062646931,-5.));
#9220=CARTESIAN_POINT('Ctrl Pts',(-6.16869034994484,6.0086782747727,-5.));
#9221=CARTESIAN_POINT('Ctrl Pts',(-6.12598670340816,5.94604715259802,-5.));
#9222=CARTESIAN_POINT('Ctrl Pts',(-6.06863042059311,5.89037560471066,-5.));
#9223=CARTESIAN_POINT('',(-4.62971553586298,4.49372618847532,-5.));
#9224=CARTESIAN_POINT('',(-6.06863042059311,5.89037560471066,-5.));
#9225=CARTESIAN_POINT('',(-4.51042861629926,3.1977921597985,-5.));
#9226=CARTESIAN_POINT('Origin',(-5.32620517920381,3.77615934370128,-5.));
#9227=CARTESIAN_POINT('',(-5.02458355455783,2.30724968377221,-5.));
#9228=CARTESIAN_POINT('Origin',(0.,0.,-5.));
#9229=CARTESIAN_POINT('',(-6.20653880480254,1.76258817211517,-5.));
#9230=CARTESIAN_POINT('Origin',(-5.93335250998519,2.72454931910811,-5.));
#9231=CARTESIAN_POINT('',(-8.13553012180811,2.31040030805735,-5.));
#9232=CARTESIAN_POINT('',(-6.20653880480254,1.76258817211517,-5.));
#9233=CARTESIAN_POINT('Ctrl Pts',(-8.13553012180811,2.31040030805735,-5.));
#9234=CARTESIAN_POINT('Ctrl Pts',(-8.28877366675838,2.35391977490952,-5.));
#9235=CARTESIAN_POINT('Ctrl Pts',(-8.45370244016016,2.34276955340629,-5.));
#9236=CARTESIAN_POINT('Ctrl Pts',(-8.6589510005022,2.33262178500855,-5.));
#9237=CARTESIAN_POINT('Ctrl Pts',(-8.83674992145663,2.32270547079067,-5.));
#9238=CARTESIAN_POINT('Ctrl Pts',(-9.28376031550984,2.23106772742646,-5.));
#9239=CARTESIAN_POINT('Ctrl Pts',(-9.63334698685098,2.14775617318178,-5.));
#9240=CARTESIAN_POINT('Ctrl Pts',(-10.7093635523845,1.67464016651609,-5.));
#9241=CARTESIAN_POINT('Ctrl Pts',(-11.3511826735682,1.26687710279248,-5.));
#9242=CARTESIAN_POINT('Ctrl Pts',(-11.9792754136349,0.704954299427533,-5.));
#9243=CARTESIAN_POINT('Origin',(0.,0.,-6.));
#9244=CARTESIAN_POINT('',(3.5,-6.06217782649107,-6.));
#9245=CARTESIAN_POINT('Origin',(0.,0.,-6.));
#9246=CARTESIAN_POINT('',(3.5,-6.06217782649107,-12.));
#9247=CARTESIAN_POINT('',(3.5,-6.06217782649107,-6.));
#9248=CARTESIAN_POINT('Origin',(0.,0.,-12.));
#9249=CARTESIAN_POINT('Origin',(0.,0.,-12.));
#9250=CARTESIAN_POINT('Origin',(0.,0.,-5.));
#9251=CARTESIAN_POINT('',(-6.75,11.6913429510899,-6.));
#9252=CARTESIAN_POINT('',(-6.75,11.6913429510899,-5.));
#9253=CARTESIAN_POINT('Origin',(0.,0.,-6.));
#9254=CARTESIAN_POINT('Origin',(0.,0.,-6.));
#9255=CARTESIAN_POINT('Origin',(0.,0.,-5.));
#9256=CARTESIAN_POINT('',(-4.51042861629926,3.1977921597985,1.5));
#9257=CARTESIAN_POINT('',(-4.51042861629926,3.1977921597985,-5.));
#9258=CARTESIAN_POINT('',(-5.02458355455783,2.30724968377221,1.5));
#9259=CARTESIAN_POINT('Origin',(0.,0.,1.5));
#9260=CARTESIAN_POINT('',(-5.02458355455783,2.30724968377221,-5.));
#9261=CARTESIAN_POINT('Origin',(-5.32620517920381,3.77615934370128,-5.));
#9262=CARTESIAN_POINT('',(-4.62971553586298,4.49372618847532,1.5));
#9263=CARTESIAN_POINT('',(-4.62971553586298,4.49372618847532,-5.));
#9264=CARTESIAN_POINT('Origin',(-5.32620517920381,3.77615934370128,1.5));
#9265=CARTESIAN_POINT('Origin',(-6.06863042059311,5.89037560471066,-5.));
#9266=CARTESIAN_POINT('',(-6.06863042059311,5.89037560471066,1.5));
#9267=CARTESIAN_POINT('',(-6.06863042059311,5.89037560471066,-5.));
#9268=CARTESIAN_POINT('',(-6.06863042059311,5.89037560471066,1.5));
#9269=CARTESIAN_POINT('Ctrl Pts',(-6.60014603862877,10.0218796774244,-5.));
#9270=CARTESIAN_POINT('Ctrl Pts',(-6.60014603862877,10.0218796774244,2.8));
#9271=CARTESIAN_POINT('Ctrl Pts',(-6.70554322746249,9.51813553829505,-5.));
#9272=CARTESIAN_POINT('Ctrl Pts',(-6.70554322746249,9.51813553829505,2.8));
#9273=CARTESIAN_POINT('Ctrl Pts',(-6.76569828978797,9.00392020322571,-5.));
#9274=CARTESIAN_POINT('Ctrl Pts',(-6.76569828978797,9.00392020322571,2.8));
#9275=CARTESIAN_POINT('Ctrl Pts',(-6.77159007596056,7.82431314720816,-5.));
#9276=CARTESIAN_POINT('Ctrl Pts',(-6.77159007596056,7.82431314720816,2.8));
#9277=CARTESIAN_POINT('Ctrl Pts',(-6.67739020638207,7.34654057751468,-5.));
#9278=CARTESIAN_POINT('Ctrl Pts',(-6.67739020638207,7.34654057751468,2.8));
#9279=CARTESIAN_POINT('Ctrl Pts',(-6.48685339577862,6.58075796115043,-5.));
#9280=CARTESIAN_POINT('Ctrl Pts',(-6.48685339577862,6.58075796115043,2.8));
#9281=CARTESIAN_POINT('Ctrl Pts',(-6.33143849535641,6.28265062646931,-5.));
#9282=CARTESIAN_POINT('Ctrl Pts',(-6.33143849535641,6.28265062646931,2.8));
#9283=CARTESIAN_POINT('Ctrl Pts',(-6.16869034994484,6.0086782747727,-5.));
#9284=CARTESIAN_POINT('Ctrl Pts',(-6.16869034994484,6.0086782747727,2.8));
#9285=CARTESIAN_POINT('Ctrl Pts',(-6.12598670340816,5.94604715259802,-5.));
#9286=CARTESIAN_POINT('Ctrl Pts',(-6.12598670340816,5.94604715259802,2.8));
#9287=CARTESIAN_POINT('Ctrl Pts',(-6.06863042059311,5.89037560471066,-5.));
#9288=CARTESIAN_POINT('Ctrl Pts',(-6.06863042059311,5.89037560471066,2.8));
#9289=CARTESIAN_POINT('Ctrl Pts',(-6.60014603862877,10.0218796774244,1.5));
#9290=CARTESIAN_POINT('Ctrl Pts',(-6.70554322746249,9.51813553829505,1.5));
#9291=CARTESIAN_POINT('Ctrl Pts',(-6.76569828978797,9.00392020322571,1.5));
#9292=CARTESIAN_POINT('Ctrl Pts',(-6.77159007596056,7.82431314720816,1.5));
#9293=CARTESIAN_POINT('Ctrl Pts',(-6.67739020638207,7.34654057751468,1.5));
#9294=CARTESIAN_POINT('Ctrl Pts',(-6.48685339577862,6.58075796115043,1.5));
#9295=CARTESIAN_POINT('Ctrl Pts',(-6.33143849535641,6.28265062646931,1.5));
#9296=CARTESIAN_POINT('Ctrl Pts',(-6.16869034994484,6.0086782747727,1.5));
#9297=CARTESIAN_POINT('Ctrl Pts',(-6.12598670340816,5.94604715259802,1.5));
#9298=CARTESIAN_POINT('Ctrl Pts',(-6.06863042059311,5.89037560471066,1.5));
#9299=CARTESIAN_POINT('Ctrl Pts',(-8.13553012180811,2.31040030805735,-5.));
#9300=CARTESIAN_POINT('Ctrl Pts',(-8.13553012180811,2.31040030805735,2.8));
#9301=CARTESIAN_POINT('Ctrl Pts',(-8.28877366675838,2.35391977490952,-5.));
#9302=CARTESIAN_POINT('Ctrl Pts',(-8.28877366675838,2.35391977490952,2.8));
#9303=CARTESIAN_POINT('Ctrl Pts',(-8.45370244016016,2.34276955340629,-5.));
#9304=CARTESIAN_POINT('Ctrl Pts',(-8.45370244016016,2.34276955340629,2.8));
#9305=CARTESIAN_POINT('Ctrl Pts',(-8.6589510005022,2.33262178500855,-5.));
#9306=CARTESIAN_POINT('Ctrl Pts',(-8.6589510005022,2.33262178500855,2.8));
#9307=CARTESIAN_POINT('Ctrl Pts',(-8.83674992145663,2.32270547079067,-5.));
#9308=CARTESIAN_POINT('Ctrl Pts',(-8.83674992145663,2.32270547079067,2.8));
#9309=CARTESIAN_POINT('Ctrl Pts',(-9.28376031550984,2.23106772742646,-5.));
#9310=CARTESIAN_POINT('Ctrl Pts',(-9.28376031550984,2.23106772742646,2.8));
#9311=CARTESIAN_POINT('Ctrl Pts',(-9.63334698685098,2.14775617318178,-5.));
#9312=CARTESIAN_POINT('Ctrl Pts',(-9.63334698685098,2.14775617318178,2.8));
#9313=CARTESIAN_POINT('Ctrl Pts',(-10.7093635523845,1.67464016651609,-5.));
#9314=CARTESIAN_POINT('Ctrl Pts',(-10.7093635523845,1.67464016651609,2.8));
#9315=CARTESIAN_POINT('Ctrl Pts',(-11.3511826735682,1.26687710279248,-5.));
#9316=CARTESIAN_POINT('Ctrl Pts',(-11.3511826735682,1.26687710279248,2.8));
#9317=CARTESIAN_POINT('Ctrl Pts',(-11.9792754136349,0.704954299427533,-5.));
#9318=CARTESIAN_POINT('Ctrl Pts',(-11.9792754136349,0.704954299427533,2.8));
#9319=CARTESIAN_POINT('',(-8.13553012180811,2.31040030805735,1.5));
#9320=CARTESIAN_POINT('',(-8.13553012180811,2.31040030805735,-5.));
#9321=CARTESIAN_POINT('Ctrl Pts',(-8.13553012180811,2.31040030805735,1.5));
#9322=CARTESIAN_POINT('Ctrl Pts',(-8.28877366675838,2.35391977490952,1.5));
#9323=CARTESIAN_POINT('Ctrl Pts',(-8.45370244016016,2.34276955340629,1.5));
#9324=CARTESIAN_POINT('Ctrl Pts',(-8.6589510005022,2.33262178500855,1.5));
#9325=CARTESIAN_POINT('Ctrl Pts',(-8.83674992145663,2.32270547079067,1.5));
#9326=CARTESIAN_POINT('Ctrl Pts',(-9.28376031550984,2.23106772742646,1.5));
#9327=CARTESIAN_POINT('Ctrl Pts',(-9.63334698685098,2.14775617318178,1.5));
#9328=CARTESIAN_POINT('Ctrl Pts',(-10.7093635523845,1.67464016651609,1.5));
#9329=CARTESIAN_POINT('Ctrl Pts',(-11.3511826735682,1.26687710279248,1.5));
#9330=CARTESIAN_POINT('Ctrl Pts',(-11.9792754136349,0.704954299427533,1.5));
#9331=CARTESIAN_POINT('Origin',(-6.20653880480254,1.76258817211517,-5.));
#9332=CARTESIAN_POINT('',(-6.20653880480254,1.76258817211517,1.5));
#9333=CARTESIAN_POINT('',(-6.20653880480254,1.76258817211517,-5.));
#9334=CARTESIAN_POINT('',(-6.20653880480254,1.76258817211517,1.5));
#9335=CARTESIAN_POINT('Origin',(-5.93335250998519,2.72454931910811,-5.));
#9336=CARTESIAN_POINT('Origin',(-5.93335250998519,2.72454931910811,1.5));
#9337=CARTESIAN_POINT('Origin',(-8.72244267930302,4.37908846803365,1.5));
#9338=CARTESIAN_POINT('Origin',(0.,0.,-5.));
#9339=CARTESIAN_POINT('',(5.02458355455784,2.3072496837722,1.5));
#9340=CARTESIAN_POINT('',(5.02458355455784,2.3072496837722,-5.));
#9341=CARTESIAN_POINT('',(4.51042861629926,3.1977921597985,1.5));
#9342=CARTESIAN_POINT('Origin',(0.,0.,1.5));
#9343=CARTESIAN_POINT('',(4.51042861629926,3.1977921597985,-5.));
#9344=CARTESIAN_POINT('Origin',(5.93335250998519,2.72454931910811,-5.));
#9345=CARTESIAN_POINT('',(6.20653880480254,1.76258817211517,1.5));
#9346=CARTESIAN_POINT('',(6.20653880480254,1.76258817211517,-5.));
#9347=CARTESIAN_POINT('Origin',(5.93335250998519,2.72454931910811,1.5));
#9348=CARTESIAN_POINT('Origin',(8.13553012180811,2.31040030805735,-5.));
#9349=CARTESIAN_POINT('',(8.13553012180811,2.31040030805735,1.5));
#9350=CARTESIAN_POINT('',(8.13553012180811,2.31040030805735,-5.));
#9351=CARTESIAN_POINT('',(8.13553012180811,2.31040030805735,1.5));
#9352=CARTESIAN_POINT('Ctrl Pts',(11.9792754136349,0.704954299427528,-5.));
#9353=CARTESIAN_POINT('Ctrl Pts',(11.9792754136349,0.704954299427528,2.8));
#9354=CARTESIAN_POINT('Ctrl Pts',(11.5957187866216,1.04810301195305,-5.));
#9355=CARTESIAN_POINT('Ctrl Pts',(11.5957187866216,1.04810301195305,2.8));
#9356=CARTESIAN_POINT('Ctrl Pts',(11.1804727745766,1.35730649166136,-5.));
#9357=CARTESIAN_POINT('Ctrl Pts',(11.1804727745766,1.35730649166136,2.8));
#9358=CARTESIAN_POINT('Ctrl Pts',(10.1618489906858,1.95221245615685,-5.));
#9359=CARTESIAN_POINT('Ctrl Pts',(10.1618489906858,1.95221245615685,2.8));
#9360=CARTESIAN_POINT('Ctrl Pts',(9.70098587343182,2.10951926090029,-5.));
#9361=CARTESIAN_POINT('Ctrl Pts',(9.70098587343182,2.10951926090029,2.8));
#9362=CARTESIAN_POINT('Ctrl Pts',(8.94253026837877,2.32740085079939,-5.));
#9363=CARTESIAN_POINT('Ctrl Pts',(8.94253026837877,2.32740085079939,2.8));
#9364=CARTESIAN_POINT('Ctrl Pts',(8.60665429329664,2.34186126624275,-5.));
#9365=CARTESIAN_POINT('Ctrl Pts',(8.60665429329664,2.34186126624275,2.8));
#9366=CARTESIAN_POINT('Ctrl Pts',(8.28801320409168,2.33790341374574,-5.));
#9367=CARTESIAN_POINT('Ctrl Pts',(8.28801320409168,2.33790341374574,2.8));
#9368=CARTESIAN_POINT('Ctrl Pts',(8.21242123795344,2.33223653209797,-5.));
#9369=CARTESIAN_POINT('Ctrl Pts',(8.21242123795344,2.33223653209797,2.8));
#9370=CARTESIAN_POINT('Ctrl Pts',(8.13553012180811,2.31040030805735,-5.));
#9371=CARTESIAN_POINT('Ctrl Pts',(8.13553012180811,2.31040030805735,2.8));
#9372=CARTESIAN_POINT('Ctrl Pts',(11.9792754136349,0.704954299427528,1.5));
#9373=CARTESIAN_POINT('Ctrl Pts',(11.5957187866216,1.04810301195305,1.5));
#9374=CARTESIAN_POINT('Ctrl Pts',(11.1804727745766,1.35730649166136,1.5));
#9375=CARTESIAN_POINT('Ctrl Pts',(10.1618489906858,1.95221245615685,1.5));
#9376=CARTESIAN_POINT('Ctrl Pts',(9.70098587343182,2.10951926090029,1.5));
#9377=CARTESIAN_POINT('Ctrl Pts',(8.94253026837877,2.32740085079939,1.5));
#9378=CARTESIAN_POINT('Ctrl Pts',(8.60665429329664,2.34186126624275,1.5));
#9379=CARTESIAN_POINT('Ctrl Pts',(8.28801320409168,2.33790341374574,1.5));
#9380=CARTESIAN_POINT('Ctrl Pts',(8.21242123795344,2.33223653209797,1.5));
#9381=CARTESIAN_POINT('Ctrl Pts',(8.13553012180811,2.31040030805735,1.5));
#9382=CARTESIAN_POINT('Ctrl Pts',(6.06863042059311,5.89037560471066,-5.));
#9383=CARTESIAN_POINT('Ctrl Pts',(6.06863042059311,5.89037560471066,2.8));
#9384=CARTESIAN_POINT('Ctrl Pts',(6.18294115692139,6.00132867417748,-5.));
#9385=CARTESIAN_POINT('Ctrl Pts',(6.18294115692139,6.00132867417748,2.8));
#9386=CARTESIAN_POINT('Ctrl Pts',(6.25574916854267,6.14973629251004,-5.));
#9387=CARTESIAN_POINT('Ctrl Pts',(6.25574916854267,6.14973629251004,2.8));
#9388=CARTESIAN_POINT('Ctrl Pts',(6.34958522348502,6.3325606440466,-5.));
#9389=CARTESIAN_POINT('Ctrl Pts',(6.34958522348502,6.3325606440466,2.8));
#9390=CARTESIAN_POINT('Ctrl Pts',(6.4298969039412,6.49149718347355,-5.));
#9391=CARTESIAN_POINT('Ctrl Pts',(6.4298969039412,6.49149718347355,2.8));
#9392=CARTESIAN_POINT('Ctrl Pts',(6.57404148726847,6.92443841215994,-5.));
#9393=CARTESIAN_POINT('Ctrl Pts',(6.57404148726847,6.92443841215994,2.8));
#9394=CARTESIAN_POINT('Ctrl Pts',(6.67668490053567,7.26884512749145,-5.));
#9395=CARTESIAN_POINT('Ctrl Pts',(6.67668490053567,7.26884512749145,2.8));
#9396=CARTESIAN_POINT('Ctrl Pts',(6.80496270256398,8.43726081120601,-5.));
#9397=CARTESIAN_POINT('Ctrl Pts',(6.80496270256398,8.43726081120601,2.8));
#9398=CARTESIAN_POINT('Ctrl Pts',(6.77273909133898,9.19697400660618,-5.));
#9399=CARTESIAN_POINT('Ctrl Pts',(6.77273909133898,9.19697400660618,2.8));
#9400=CARTESIAN_POINT('Ctrl Pts',(6.60014603862878,10.0218796774244,-5.));
#9401=CARTESIAN_POINT('Ctrl Pts',(6.60014603862878,10.0218796774244,2.8));
#9402=CARTESIAN_POINT('',(6.06863042059311,5.89037560471066,1.5));
#9403=CARTESIAN_POINT('',(6.06863042059311,5.89037560471066,-5.));
#9404=CARTESIAN_POINT('Ctrl Pts',(6.06863042059311,5.89037560471066,1.5));
#9405=CARTESIAN_POINT('Ctrl Pts',(6.18294115692139,6.00132867417748,1.5));
#9406=CARTESIAN_POINT('Ctrl Pts',(6.25574916854267,6.14973629251004,1.5));
#9407=CARTESIAN_POINT('Ctrl Pts',(6.34958522348502,6.3325606440466,1.5));
#9408=CARTESIAN_POINT('Ctrl Pts',(6.4298969039412,6.49149718347355,1.5));
#9409=CARTESIAN_POINT('Ctrl Pts',(6.57404148726847,6.92443841215994,1.5));
#9410=CARTESIAN_POINT('Ctrl Pts',(6.67668490053567,7.26884512749145,1.5));
#9411=CARTESIAN_POINT('Ctrl Pts',(6.80496270256398,8.43726081120601,1.5));
#9412=CARTESIAN_POINT('Ctrl Pts',(6.77273909133898,9.19697400660618,1.5));
#9413=CARTESIAN_POINT('Ctrl Pts',(6.60014603862878,10.0218796774244,1.5));
#9414=CARTESIAN_POINT('Origin',(4.62971553586298,4.49372618847532,-5.));
#9415=CARTESIAN_POINT('',(4.62971553586298,4.49372618847532,1.5));
#9416=CARTESIAN_POINT('',(4.62971553586298,4.49372618847532,-5.));
#9417=CARTESIAN_POINT('',(4.62971553586298,4.49372618847532,1.5));
#9418=CARTESIAN_POINT('Origin',(5.32620517920381,3.77615934370128,-5.));
#9419=CARTESIAN_POINT('Origin',(5.32620517920381,3.77615934370128,1.5));
#9420=CARTESIAN_POINT('Origin',(7.57758128266783,4.37595288274577,1.5));
#9421=CARTESIAN_POINT('Origin',(0.,0.,-5.));
#9422=CARTESIAN_POINT('',(-0.51415493825858,-5.5050418435707,1.5));
#9423=CARTESIAN_POINT('',(-0.51415493825858,-5.5050418435707,-5.));
#9424=CARTESIAN_POINT('',(0.514154938258578,-5.5050418435707,1.5));
#9425=CARTESIAN_POINT('Origin',(0.,0.,1.5));
#9426=CARTESIAN_POINT('',(0.514154938258578,-5.5050418435707,-5.));
#9427=CARTESIAN_POINT('Origin',(-0.607147330781382,-6.50070866280939,-5.));
#9428=CARTESIAN_POINT('',(-1.57682326893956,-6.25631436059049,1.5));
#9429=CARTESIAN_POINT('',(-1.57682326893956,-6.25631436059049,-5.));
#9430=CARTESIAN_POINT('Origin',(-0.607147330781382,-6.50070866280939,1.5));
#9431=CARTESIAN_POINT('Origin',(-2.06689970121501,-8.20077591276801,-5.));
#9432=CARTESIAN_POINT('',(-2.06689970121501,-8.20077591276801,1.5));
#9433=CARTESIAN_POINT('',(-2.06689970121501,-8.20077591276801,-5.));
#9434=CARTESIAN_POINT('',(-2.06689970121501,-8.20077591276801,1.5));
#9435=CARTESIAN_POINT('Ctrl Pts',(-5.37912937500618,-10.726833976852,-5.));
#9436=CARTESIAN_POINT('Ctrl Pts',(-5.37912937500618,-10.726833976852,2.8));
#9437=CARTESIAN_POINT('Ctrl Pts',(-4.89017555905846,-10.5662385502925,-5.));
#9438=CARTESIAN_POINT('Ctrl Pts',(-4.89017555905846,-10.5662385502925,2.8));
#9439=CARTESIAN_POINT('Ctrl Pts',(-4.41477448471897,-10.3612266948947,-5.));
#9440=CARTESIAN_POINT('Ctrl Pts',(-4.41477448471897,-10.3612266948947,2.8));
#9441=CARTESIAN_POINT('Ctrl Pts',(-3.39025891465935,-9.77652560339542,-5.));
#9442=CARTESIAN_POINT('Ctrl Pts',(-3.39025891465935,-9.77652560339542,2.8));
#9443=CARTESIAN_POINT('Ctrl Pts',(-3.02359566682149,-9.45605983842045,-5.));
#9444=CARTESIAN_POINT('Ctrl Pts',(-3.02359566682149,-9.45605983842045,2.8));
#9445=CARTESIAN_POINT('Ctrl Pts',(-2.45567687261362,-8.90815881193254,-5.));
#9446=CARTESIAN_POINT('Ctrl Pts',(-2.45567687261362,-8.90815881193254,2.8));
#9447=CARTESIAN_POINT('Ctrl Pts',(-2.27521579794306,-8.62451189270596,-5.));
#9448=CARTESIAN_POINT('Ctrl Pts',(-2.27521579794306,-8.62451189270596,2.8));
#9449=CARTESIAN_POINT('Ctrl Pts',(-2.11932285414849,-8.34658168851868,-5.));
#9450=CARTESIAN_POINT('Ctrl Pts',(-2.11932285414849,-8.34658168851868,2.8));
#9451=CARTESIAN_POINT('Ctrl Pts',(-2.0864345345459,-8.27828368469604,-5.));
#9452=CARTESIAN_POINT('Ctrl Pts',(-2.0864345345459,-8.27828368469604,2.8));
#9453=CARTESIAN_POINT('Ctrl Pts',(-2.06689970121501,-8.20077591276801,-5.));
#9454=CARTESIAN_POINT('Ctrl Pts',(-2.06689970121501,-8.20077591276801,2.8));
#9455=CARTESIAN_POINT('',(-5.37912937500618,-10.726833976852,1.5));
#9456=CARTESIAN_POINT('',(-5.37912937500618,-10.726833976852,-5.));
#9457=CARTESIAN_POINT('Ctrl Pts',(-5.37912937500618,-10.726833976852,1.5));
#9458=CARTESIAN_POINT('Ctrl Pts',(-4.89017555905846,-10.5662385502925,1.5));
#9459=CARTESIAN_POINT('Ctrl Pts',(-4.41477448471897,-10.3612266948947,1.5));
#9460=CARTESIAN_POINT('Ctrl Pts',(-3.39025891465935,-9.77652560339542,1.5));
#9461=CARTESIAN_POINT('Ctrl Pts',(-3.02359566682149,-9.45605983842045,1.5));
#9462=CARTESIAN_POINT('Ctrl Pts',(-2.45567687261362,-8.90815881193254,1.5));
#9463=CARTESIAN_POINT('Ctrl Pts',(-2.27521579794306,-8.62451189270596,1.5));
#9464=CARTESIAN_POINT('Ctrl Pts',(-2.11932285414849,-8.34658168851868,1.5));
#9465=CARTESIAN_POINT('Ctrl Pts',(-2.0864345345459,-8.27828368469604,1.5));
#9466=CARTESIAN_POINT('Ctrl Pts',(-2.06689970121501,-8.20077591276801,1.5));
#9467=CARTESIAN_POINT('Origin',(0.,0.,-5.));
#9468=CARTESIAN_POINT('',(5.37912937500617,-10.726833976852,1.5));
#9469=CARTESIAN_POINT('',(5.37912937500617,-10.726833976852,-5.));
#9470=CARTESIAN_POINT('Origin',(0.,0.,1.5));
#9471=CARTESIAN_POINT('Ctrl Pts',(2.066899701215,-8.20077591276801,-5.));
#9472=CARTESIAN_POINT('Ctrl Pts',(2.066899701215,-8.20077591276801,2.8));
#9473=CARTESIAN_POINT('Ctrl Pts',(2.105832509837,-8.35524844908701,-5.));
#9474=CARTESIAN_POINT('Ctrl Pts',(2.105832509837,-8.35524844908701,2.8));
#9475=CARTESIAN_POINT('Ctrl Pts',(2.19795327161749,-8.49250584591635,-5.));
#9476=CARTESIAN_POINT('Ctrl Pts',(2.19795327161749,-8.49250584591635,2.8));
#9477=CARTESIAN_POINT('Ctrl Pts',(2.30936577701074,-8.66518242906081,-5.));
#9478=CARTESIAN_POINT('Ctrl Pts',(2.30936577701074,-8.66518242906081,2.8));
#9479=CARTESIAN_POINT('Ctrl Pts',(2.40685301751416,-8.81420265426653,-5.));
#9480=CARTESIAN_POINT('Ctrl Pts',(2.40685301751416,-8.81420265426653,2.8));
#9481=CARTESIAN_POINT('Ctrl Pts',(2.70971882824218,-9.15550613959305,-5.));
#9482=CARTESIAN_POINT('Ctrl Pts',(2.70971882824218,-9.15550613959305,2.8));
#9483=CARTESIAN_POINT('Ctrl Pts',(2.95666208631803,-9.41660130067616,-5.));
#9484=CARTESIAN_POINT('Ctrl Pts',(2.95666208631803,-9.41660130067616,2.8));
#9485=CARTESIAN_POINT('Ctrl Pts',(3.90440084969946,-10.1119009779187,-5.));
#9486=CARTESIAN_POINT('Ctrl Pts',(3.90440084969946,-10.1119009779187,2.8));
#9487=CARTESIAN_POINT('Ctrl Pts',(4.57844358216429,-10.4638511096618,-5.));
#9488=CARTESIAN_POINT('Ctrl Pts',(4.57844358216429,-10.4638511096618,2.8));
#9489=CARTESIAN_POINT('Ctrl Pts',(5.37912937500617,-10.726833976852,-5.));
#9490=CARTESIAN_POINT('Ctrl Pts',(5.37912937500617,-10.726833976852,2.8));
#9491=CARTESIAN_POINT('',(2.066899701215,-8.20077591276801,1.5));
#9492=CARTESIAN_POINT('',(2.066899701215,-8.20077591276801,-5.));
#9493=CARTESIAN_POINT('Ctrl Pts',(2.066899701215,-8.20077591276801,1.5));
#9494=CARTESIAN_POINT('Ctrl Pts',(2.105832509837,-8.35524844908701,1.5));
#9495=CARTESIAN_POINT('Ctrl Pts',(2.19795327161749,-8.49250584591635,1.5));
#9496=CARTESIAN_POINT('Ctrl Pts',(2.30936577701074,-8.66518242906081,1.5));
#9497=CARTESIAN_POINT('Ctrl Pts',(2.40685301751416,-8.81420265426653,1.5));
#9498=CARTESIAN_POINT('Ctrl Pts',(2.70971882824218,-9.15550613959305,1.5));
#9499=CARTESIAN_POINT('Ctrl Pts',(2.95666208631803,-9.41660130067616,1.5));
#9500=CARTESIAN_POINT('Ctrl Pts',(3.90440084969946,-10.1119009779187,1.5));
#9501=CARTESIAN_POINT('Ctrl Pts',(4.57844358216429,-10.4638511096618,1.5));
#9502=CARTESIAN_POINT('Ctrl Pts',(5.37912937500617,-10.726833976852,1.5));
#9503=CARTESIAN_POINT('Origin',(1.57682326893955,-6.25631436059049,-5.));
#9504=CARTESIAN_POINT('',(1.57682326893955,-6.25631436059049,1.5));
#9505=CARTESIAN_POINT('',(1.57682326893955,-6.25631436059049,-5.));
#9506=CARTESIAN_POINT('',(1.57682326893955,-6.25631436059049,1.5));
#9507=CARTESIAN_POINT('Origin',(0.607147330781379,-6.50070866280939,-5.));
#9508=CARTESIAN_POINT('Origin',(0.607147330781379,-6.50070866280939,1.5));
#9509=CARTESIAN_POINT('Origin',(-0.566820186385169,-9.74328117350263,1.5));
#9804=UNCERTAINTY_MEASURE_WITH_UNIT(LENGTH_MEASURE(0.01),#9823,
'DISTANCE_ACCURACY_VALUE',
'Maximum model space distance between geometric entities at asserted c
onnectivities');
#9811=UNCERTAINTY_MEASURE_WITH_UNIT(LENGTH_MEASURE(0.01),#9823,
'DISTANCE_ACCURACY_VALUE',
'Maximum model space distance between geometric entities at asserted c
onnectivities');
#9815=(
GEOMETRIC_REPRESENTATION_CONTEXT(3)
GLOBAL_UNCERTAINTY_ASSIGNED_CONTEXT((#9804))
GLOBAL_UNIT_ASSIGNED_CONTEXT((#9823,#9825,#9826))
REPRESENTATION_CONTEXT('','3D')
);
#9822=(
GEOMETRIC_REPRESENTATION_CONTEXT(3)
GLOBAL_UNCERTAINTY_ASSIGNED_CONTEXT((#9811))
GLOBAL_UNIT_ASSIGNED_CONTEXT((#9823,#9825,#9826))
REPRESENTATION_CONTEXT('','3D')
);
#9823=(
LENGTH_UNIT()
NAMED_UNIT(*)
SI_UNIT(.MILLI.,.METRE.)
);
#9825=(
NAMED_UNIT(*)
PLANE_ANGLE_UNIT()
SI_UNIT($,.RADIAN.)
);
#9826=(
NAMED_UNIT(*)
SI_UNIT($,.STERADIAN.)
SOLID_ANGLE_UNIT()
);
#9830=SHAPE_DEFINITION_REPRESENTATION(#9840,#9859);
#9840=PRODUCT_DEFINITION_SHAPE('',$,#9870);
#9859=SHAPE_REPRESENTATION('',(#3566),#9815);
#9866=PRODUCT_DEFINITION_CONTEXT('part definition',#9898,'design');
#9870=PRODUCT_DEFINITION('Hub_02','Hub_02',#9880,#9866);
#9880=PRODUCT_DEFINITION_FORMATION('',$,#9903);
#9898=APPLICATION_CONTEXT(
'Core Data for Automotive Mechanical Design Process');
#9899=PRODUCT_CONTEXT('part definition',#9898,'mechanical');
#9903=PRODUCT('Hub_02','Hub_02',$,(#9899));
#9911=PRESENTATION_STYLE_ASSIGNMENT((#9914));
#9914=SURFACE_STYLE_USAGE(.BOTH.,#9917);
#9917=SURFACE_SIDE_STYLE('',(#9920));
#9920=SURFACE_STYLE_FILL_AREA(#9923);
#9923=FILL_AREA_STYLE('Opaque(78,78,78)',(#9926));
#9926=FILL_AREA_STYLE_COLOUR('Opaque(78,78,78)',#9929);
#9929=COLOUR_RGB('Opaque(78,78,78)', 0.09019608, 0.27058824, 0.51372549);
ENDSEC;
END-ISO-10303-21;
